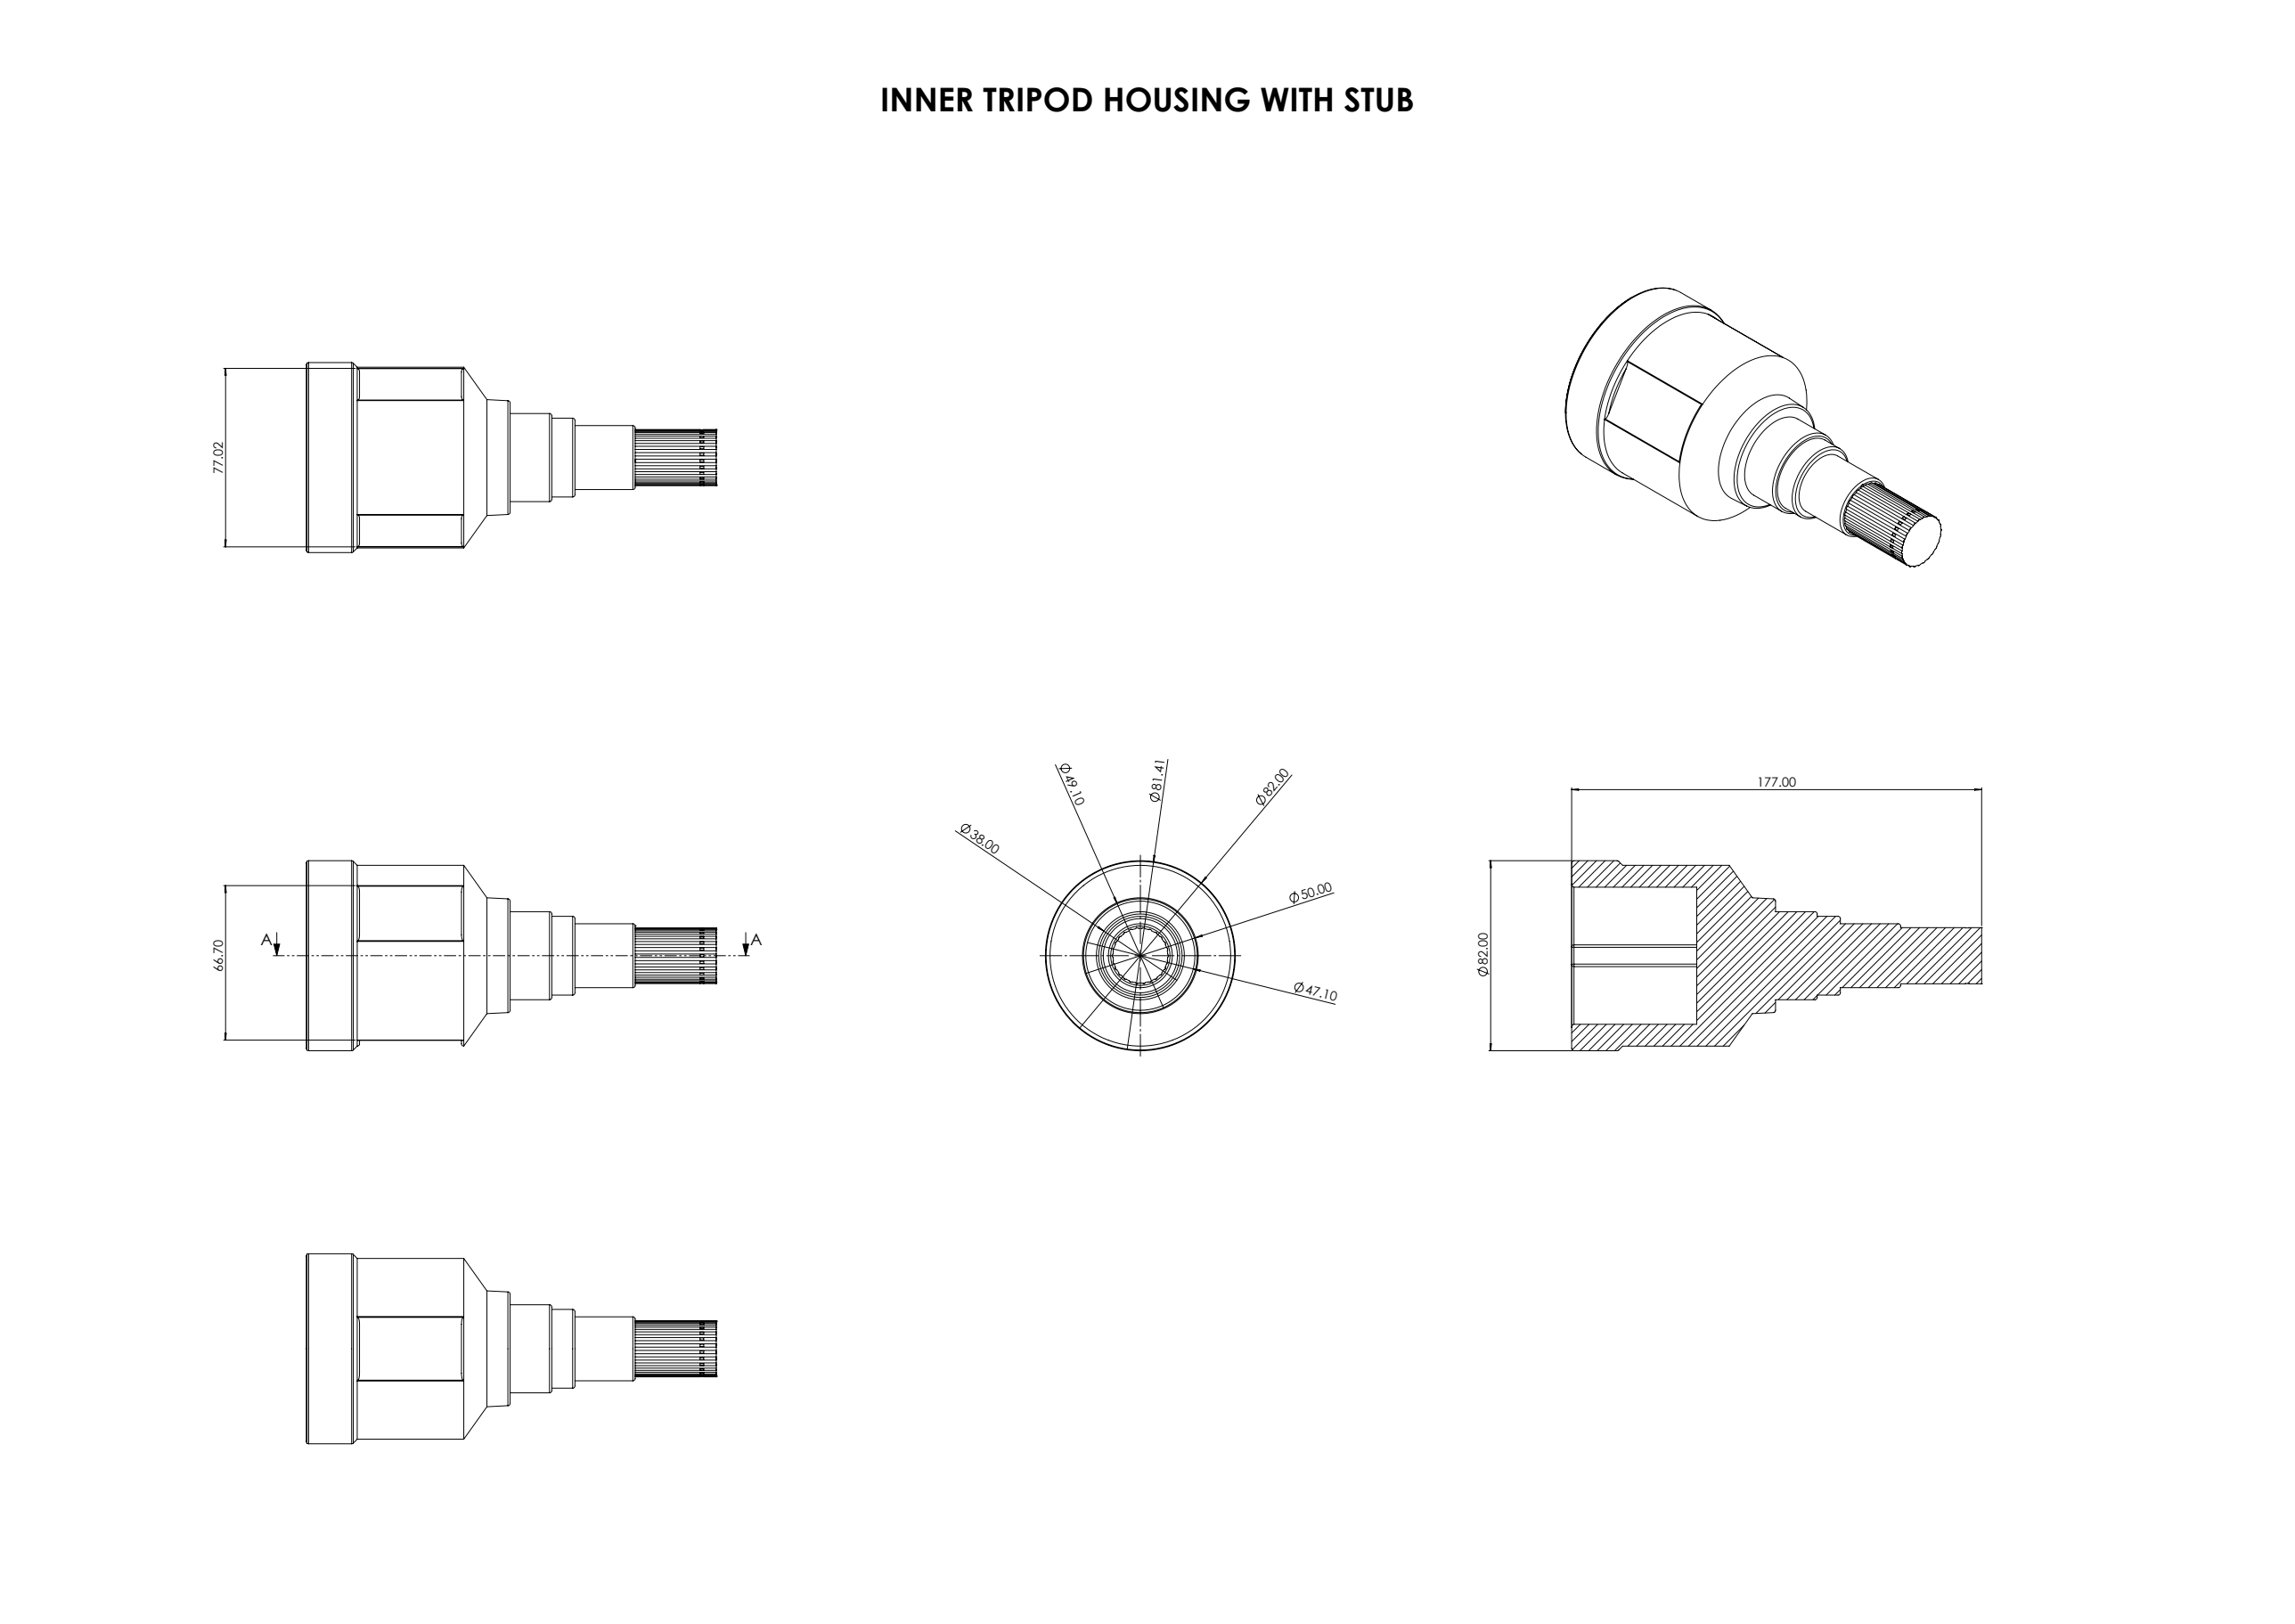
ISO-10303-21;
HEADER;
/* Generated by software containing ST-Developer
 * from STEP Tools, Inc. (www.steptools.com) 
 */

FILE_DESCRIPTION(
/* description */ (''),
/* implementation_level */ '2;1');

FILE_NAME(
/* name */ '13_Inner_Tripod_Housing_with_Stub.step',
/* time_stamp */ '2026-10-11T12:57:03-07:00',
/* author */ (''),
/* organization */ (''),
/* preprocessor_version */ 'ST-DEVELOPER v20.2',
/* originating_system */ 'Autodesk Translation Framework v15.15.0.0',
/* authorisation */ '');

FILE_SCHEMA (('AUTOMOTIVE_DESIGN { 1 0 10303 214 3 1 1 }'));
ENDSEC;

DATA;
#10=MECHANICAL_DESIGN_GEOMETRIC_PRESENTATION_REPRESENTATION('',(#268),#90374);
#234=SHAPE_REPRESENTATION_RELATIONSHIP('SRR','None',#90453,#251);
#251=ADVANCED_BREP_SHAPE_REPRESENTATION('',(#285),#90369);
#268=STYLED_ITEM('',(#90666),#285);
#285=MANIFOLD_SOLID_BREP('Body1',#40357);
#567=SPHERICAL_SURFACE('',#44329,1.);
#568=SPHERICAL_SURFACE('',#44334,1.);
#569=SPHERICAL_SURFACE('',#44356,1.);
#570=SPHERICAL_SURFACE('',#44371,1.);
#571=SPHERICAL_SURFACE('',#44381,1.);
#572=SPHERICAL_SURFACE('',#44386,1.);
#745=CONICAL_SURFACE('',#44294,24.75,0.0499583957219426);
#746=CONICAL_SURFACE('',#44306,40.,0.785398163397441);
#747=CONICAL_SURFACE('',#44318,40.7,0.785398163397426);
#748=CONICAL_SURFACE('',#44512,12.5,0.785398163397459);
#749=CONICAL_SURFACE('',#44524,12.5,0.785398163397459);
#750=CONICAL_SURFACE('',#44534,12.5,0.785398163397459);
#751=CONICAL_SURFACE('',#44544,12.5,0.785398163397459);
#752=CONICAL_SURFACE('',#44554,12.5,0.785398163397459);
#753=CONICAL_SURFACE('',#44564,12.5,0.785398163397459);
#754=CONICAL_SURFACE('',#44574,12.5,0.785398163397459);
#755=CONICAL_SURFACE('',#44584,12.5,0.785398163397459);
#756=CONICAL_SURFACE('',#44594,12.5,0.785398163397459);
#757=CONICAL_SURFACE('',#44604,12.5,0.785398163397459);
#758=CONICAL_SURFACE('',#44614,12.5,0.785398163397459);
#759=CONICAL_SURFACE('',#44624,12.5,0.785398163397459);
#760=CONICAL_SURFACE('',#44634,12.5,0.785398163397459);
#761=CONICAL_SURFACE('',#44644,12.5,0.785398163397459);
#762=CONICAL_SURFACE('',#44654,12.5,0.785398163397459);
#763=CONICAL_SURFACE('',#44664,12.5,0.785398163397459);
#764=CONICAL_SURFACE('',#44674,12.5,0.785398163397459);
#765=CONICAL_SURFACE('',#44684,12.5,0.785398163397459);
#766=CONICAL_SURFACE('',#44694,12.5,0.785398163397459);
#767=CONICAL_SURFACE('',#44704,12.5,0.785398163397459);
#768=CONICAL_SURFACE('',#44714,12.5,0.785398163397459);
#769=CONICAL_SURFACE('',#44724,12.5,0.785398163397459);
#770=CONICAL_SURFACE('',#44734,12.5,0.785398163397459);
#771=CONICAL_SURFACE('',#44744,12.5,0.785398163397459);
#772=CONICAL_SURFACE('',#44750,12.5,0.785398163397459);
#773=CONICAL_SURFACE('',#44773,12.5,0.785398163397459);
#774=CONICAL_SURFACE('',#44807,32.,0.950546840812075);
#991=TOROIDAL_SURFACE('',#44272,16.,1.);
#992=TOROIDAL_SURFACE('',#44281,18.,1.);
#993=TOROIDAL_SURFACE('',#44289,23.548750780275,1.);
#994=TOROIDAL_SURFACE('',#44297,40.,1.);
#995=TOROIDAL_SURFACE('',#44314,40.,1.);
#996=TOROIDAL_SURFACE('',#44324,16.5,1.);
#997=TOROIDAL_SURFACE('',#44339,19.,1.);
#998=TOROIDAL_SURFACE('',#44348,19.,1.);
#999=TOROIDAL_SURFACE('',#44361,16.5,1.);
#1000=TOROIDAL_SURFACE('',#44363,39.9857864376269,1.);
#1001=TOROIDAL_SURFACE('',#44373,16.5,1.);
#1002=TOROIDAL_SURFACE('',#44383,19.,1.);
#1003=TOROIDAL_SURFACE('',#44392,38.,1.);
#1004=TOROIDAL_SURFACE('',#44399,38.,1.);
#1005=TOROIDAL_SURFACE('',#44402,38.,1.);
#1006=TOROIDAL_SURFACE('',#44406,38.,1.);
#1007=TOROIDAL_SURFACE('',#44415,38.,1.);
#1008=TOROIDAL_SURFACE('',#44419,38.,1.);
#1009=TOROIDAL_SURFACE('',#44763,12.8,1.);
#1077=FACE_BOUND('',#6525,.T.);
#1078=FACE_BOUND('',#6529,.T.);
#1079=FACE_BOUND('',#6533,.T.);
#1080=FACE_BOUND('',#6547,.T.);
#1081=FACE_BOUND('',#6588,.T.);
#1082=FACE_BOUND('',#6597,.T.);
#1083=FACE_BOUND('',#6603,.T.);
#1084=FACE_BOUND('',#6609,.T.);
#1085=FACE_BOUND('',#6615,.T.);
#1086=FACE_BOUND('',#6621,.T.);
#1087=FACE_BOUND('',#6627,.T.);
#1088=FACE_BOUND('',#6633,.T.);
#1089=FACE_BOUND('',#6639,.T.);
#1090=FACE_BOUND('',#6645,.T.);
#1091=FACE_BOUND('',#6651,.T.);
#1092=FACE_BOUND('',#6657,.T.);
#1093=FACE_BOUND('',#6663,.T.);
#1094=FACE_BOUND('',#6669,.T.);
#1095=FACE_BOUND('',#6675,.T.);
#1096=FACE_BOUND('',#6681,.T.);
#1097=FACE_BOUND('',#6687,.T.);
#1098=FACE_BOUND('',#6693,.T.);
#1099=FACE_BOUND('',#6699,.T.);
#1100=FACE_BOUND('',#6705,.T.);
#1101=FACE_BOUND('',#6711,.T.);
#1102=FACE_BOUND('',#6717,.T.);
#1103=FACE_BOUND('',#6723,.T.);
#1104=FACE_BOUND('',#6729,.T.);
#1105=FACE_BOUND('',#6735,.T.);
#1106=FACE_BOUND('',#6740,.T.);
#1107=FACE_BOUND('',#6745,.T.);
#1641=PLANE('',#44279);
#1642=PLANE('',#44288);
#1643=PLANE('',#44296);
#1644=PLANE('',#44342);
#1645=PLANE('',#44366);
#1646=PLANE('',#44396);
#1647=PLANE('',#44401);
#1648=PLANE('',#44409);
#1649=PLANE('',#44410);
#1650=PLANE('',#44422);
#1651=PLANE('',#44423);
#1652=PLANE('',#44433);
#1653=PLANE('',#44434);
#1654=PLANE('',#44435);
#1655=PLANE('',#44515);
#1656=PLANE('',#44523);
#1657=PLANE('',#44525);
#1658=PLANE('',#44533);
#1659=PLANE('',#44535);
#1660=PLANE('',#44543);
#1661=PLANE('',#44545);
#1662=PLANE('',#44553);
#1663=PLANE('',#44555);
#1664=PLANE('',#44563);
#1665=PLANE('',#44565);
#1666=PLANE('',#44573);
#1667=PLANE('',#44575);
#1668=PLANE('',#44583);
#1669=PLANE('',#44585);
#1670=PLANE('',#44593);
#1671=PLANE('',#44595);
#1672=PLANE('',#44603);
#1673=PLANE('',#44605);
#1674=PLANE('',#44613);
#1675=PLANE('',#44615);
#1676=PLANE('',#44623);
#1677=PLANE('',#44625);
#1678=PLANE('',#44633);
#1679=PLANE('',#44635);
#1680=PLANE('',#44643);
#1681=PLANE('',#44645);
#1682=PLANE('',#44653);
#1683=PLANE('',#44655);
#1684=PLANE('',#44663);
#1685=PLANE('',#44665);
#1686=PLANE('',#44673);
#1687=PLANE('',#44675);
#1688=PLANE('',#44683);
#1689=PLANE('',#44685);
#1690=PLANE('',#44693);
#1691=PLANE('',#44695);
#1692=PLANE('',#44703);
#1693=PLANE('',#44705);
#1694=PLANE('',#44713);
#1695=PLANE('',#44715);
#1696=PLANE('',#44723);
#1697=PLANE('',#44725);
#1698=PLANE('',#44733);
#1699=PLANE('',#44735);
#1700=PLANE('',#44743);
#1701=PLANE('',#44745);
#1702=PLANE('',#44754);
#1703=PLANE('',#44762);
#1704=PLANE('',#44770);
#1705=PLANE('',#44774);
#1706=PLANE('',#44775);
#1707=PLANE('',#44776);
#1708=PLANE('',#44777);
#1709=PLANE('',#44778);
#1710=PLANE('',#44779);
#1711=PLANE('',#44780);
#1712=PLANE('',#44781);
#1713=PLANE('',#44782);
#1714=PLANE('',#44783);
#1715=PLANE('',#44784);
#1716=PLANE('',#44785);
#1717=PLANE('',#44786);
#1718=PLANE('',#44787);
#1719=PLANE('',#44788);
#1720=PLANE('',#44789);
#1721=PLANE('',#44790);
#1722=PLANE('',#44791);
#1723=PLANE('',#44792);
#1724=PLANE('',#44793);
#1725=PLANE('',#44794);
#1726=PLANE('',#44795);
#1727=PLANE('',#44796);
#1728=PLANE('',#44797);
#1729=PLANE('',#44798);
#1730=PLANE('',#44799);
#1731=PLANE('',#44801);
#1732=PLANE('',#44802);
#1733=PLANE('',#44803);
#1734=PLANE('',#44804);
#1735=PLANE('',#44808);
#4088=FACE_OUTER_BOUND('',#6522,.T.);
#4089=FACE_OUTER_BOUND('',#6523,.T.);
#4090=FACE_OUTER_BOUND('',#6524,.T.);
#4091=FACE_OUTER_BOUND('',#6526,.T.);
#4092=FACE_OUTER_BOUND('',#6527,.T.);
#4093=FACE_OUTER_BOUND('',#6528,.T.);
#4094=FACE_OUTER_BOUND('',#6530,.T.);
#4095=FACE_OUTER_BOUND('',#6531,.T.);
#4096=FACE_OUTER_BOUND('',#6532,.T.);
#4097=FACE_OUTER_BOUND('',#6534,.T.);
#4098=FACE_OUTER_BOUND('',#6535,.T.);
#4099=FACE_OUTER_BOUND('',#6536,.T.);
#4100=FACE_OUTER_BOUND('',#6537,.T.);
#4101=FACE_OUTER_BOUND('',#6538,.T.);
#4102=FACE_OUTER_BOUND('',#6539,.T.);
#4103=FACE_OUTER_BOUND('',#6540,.T.);
#4104=FACE_OUTER_BOUND('',#6541,.T.);
#4105=FACE_OUTER_BOUND('',#6542,.T.);
#4106=FACE_OUTER_BOUND('',#6543,.T.);
#4107=FACE_OUTER_BOUND('',#6544,.T.);
#4108=FACE_OUTER_BOUND('',#6545,.T.);
#4109=FACE_OUTER_BOUND('',#6546,.T.);
#4110=FACE_OUTER_BOUND('',#6548,.T.);
#4111=FACE_OUTER_BOUND('',#6549,.T.);
#4112=FACE_OUTER_BOUND('',#6550,.T.);
#4113=FACE_OUTER_BOUND('',#6551,.T.);
#4114=FACE_OUTER_BOUND('',#6552,.T.);
#4115=FACE_OUTER_BOUND('',#6553,.T.);
#4116=FACE_OUTER_BOUND('',#6554,.T.);
#4117=FACE_OUTER_BOUND('',#6555,.T.);
#4118=FACE_OUTER_BOUND('',#6556,.T.);
#4119=FACE_OUTER_BOUND('',#6557,.T.);
#4120=FACE_OUTER_BOUND('',#6558,.T.);
#4121=FACE_OUTER_BOUND('',#6559,.T.);
#4122=FACE_OUTER_BOUND('',#6560,.T.);
#4123=FACE_OUTER_BOUND('',#6561,.T.);
#4124=FACE_OUTER_BOUND('',#6562,.T.);
#4125=FACE_OUTER_BOUND('',#6563,.T.);
#4126=FACE_OUTER_BOUND('',#6564,.T.);
#4127=FACE_OUTER_BOUND('',#6565,.T.);
#4128=FACE_OUTER_BOUND('',#6566,.T.);
#4129=FACE_OUTER_BOUND('',#6567,.T.);
#4130=FACE_OUTER_BOUND('',#6568,.T.);
#4131=FACE_OUTER_BOUND('',#6569,.T.);
#4132=FACE_OUTER_BOUND('',#6570,.T.);
#4133=FACE_OUTER_BOUND('',#6571,.T.);
#4134=FACE_OUTER_BOUND('',#6572,.T.);
#4135=FACE_OUTER_BOUND('',#6573,.T.);
#4136=FACE_OUTER_BOUND('',#6574,.T.);
#4137=FACE_OUTER_BOUND('',#6575,.T.);
#4138=FACE_OUTER_BOUND('',#6576,.T.);
#4139=FACE_OUTER_BOUND('',#6577,.T.);
#4140=FACE_OUTER_BOUND('',#6578,.T.);
#4141=FACE_OUTER_BOUND('',#6579,.T.);
#4142=FACE_OUTER_BOUND('',#6580,.T.);
#4143=FACE_OUTER_BOUND('',#6581,.T.);
#4144=FACE_OUTER_BOUND('',#6582,.T.);
#4145=FACE_OUTER_BOUND('',#6583,.T.);
#4146=FACE_OUTER_BOUND('',#6584,.T.);
#4147=FACE_OUTER_BOUND('',#6585,.T.);
#4148=FACE_OUTER_BOUND('',#6586,.T.);
#4149=FACE_OUTER_BOUND('',#6587,.T.);
#4150=FACE_OUTER_BOUND('',#6589,.T.);
#4151=FACE_OUTER_BOUND('',#6590,.T.);
#4152=FACE_OUTER_BOUND('',#6591,.T.);
#4153=FACE_OUTER_BOUND('',#6592,.T.);
#4154=FACE_OUTER_BOUND('',#6593,.T.);
#4155=FACE_OUTER_BOUND('',#6594,.T.);
#4156=FACE_OUTER_BOUND('',#6595,.T.);
#4157=FACE_OUTER_BOUND('',#6596,.T.);
#4158=FACE_OUTER_BOUND('',#6598,.T.);
#4159=FACE_OUTER_BOUND('',#6599,.T.);
#4160=FACE_OUTER_BOUND('',#6600,.T.);
#4161=FACE_OUTER_BOUND('',#6601,.T.);
#4162=FACE_OUTER_BOUND('',#6602,.T.);
#4163=FACE_OUTER_BOUND('',#6604,.T.);
#4164=FACE_OUTER_BOUND('',#6605,.T.);
#4165=FACE_OUTER_BOUND('',#6606,.T.);
#4166=FACE_OUTER_BOUND('',#6607,.T.);
#4167=FACE_OUTER_BOUND('',#6608,.T.);
#4168=FACE_OUTER_BOUND('',#6610,.T.);
#4169=FACE_OUTER_BOUND('',#6611,.T.);
#4170=FACE_OUTER_BOUND('',#6612,.T.);
#4171=FACE_OUTER_BOUND('',#6613,.T.);
#4172=FACE_OUTER_BOUND('',#6614,.T.);
#4173=FACE_OUTER_BOUND('',#6616,.T.);
#4174=FACE_OUTER_BOUND('',#6617,.T.);
#4175=FACE_OUTER_BOUND('',#6618,.T.);
#4176=FACE_OUTER_BOUND('',#6619,.T.);
#4177=FACE_OUTER_BOUND('',#6620,.T.);
#4178=FACE_OUTER_BOUND('',#6622,.T.);
#4179=FACE_OUTER_BOUND('',#6623,.T.);
#4180=FACE_OUTER_BOUND('',#6624,.T.);
#4181=FACE_OUTER_BOUND('',#6625,.T.);
#4182=FACE_OUTER_BOUND('',#6626,.T.);
#4183=FACE_OUTER_BOUND('',#6628,.T.);
#4184=FACE_OUTER_BOUND('',#6629,.T.);
#4185=FACE_OUTER_BOUND('',#6630,.T.);
#4186=FACE_OUTER_BOUND('',#6631,.T.);
#4187=FACE_OUTER_BOUND('',#6632,.T.);
#4188=FACE_OUTER_BOUND('',#6634,.T.);
#4189=FACE_OUTER_BOUND('',#6635,.T.);
#4190=FACE_OUTER_BOUND('',#6636,.T.);
#4191=FACE_OUTER_BOUND('',#6637,.T.);
#4192=FACE_OUTER_BOUND('',#6638,.T.);
#4193=FACE_OUTER_BOUND('',#6640,.T.);
#4194=FACE_OUTER_BOUND('',#6641,.T.);
#4195=FACE_OUTER_BOUND('',#6642,.T.);
#4196=FACE_OUTER_BOUND('',#6643,.T.);
#4197=FACE_OUTER_BOUND('',#6644,.T.);
#4198=FACE_OUTER_BOUND('',#6646,.T.);
#4199=FACE_OUTER_BOUND('',#6647,.T.);
#4200=FACE_OUTER_BOUND('',#6648,.T.);
#4201=FACE_OUTER_BOUND('',#6649,.T.);
#4202=FACE_OUTER_BOUND('',#6650,.T.);
#4203=FACE_OUTER_BOUND('',#6652,.T.);
#4204=FACE_OUTER_BOUND('',#6653,.T.);
#4205=FACE_OUTER_BOUND('',#6654,.T.);
#4206=FACE_OUTER_BOUND('',#6655,.T.);
#4207=FACE_OUTER_BOUND('',#6656,.T.);
#4208=FACE_OUTER_BOUND('',#6658,.T.);
#4209=FACE_OUTER_BOUND('',#6659,.T.);
#4210=FACE_OUTER_BOUND('',#6660,.T.);
#4211=FACE_OUTER_BOUND('',#6661,.T.);
#4212=FACE_OUTER_BOUND('',#6662,.T.);
#4213=FACE_OUTER_BOUND('',#6664,.T.);
#4214=FACE_OUTER_BOUND('',#6665,.T.);
#4215=FACE_OUTER_BOUND('',#6666,.T.);
#4216=FACE_OUTER_BOUND('',#6667,.T.);
#4217=FACE_OUTER_BOUND('',#6668,.T.);
#4218=FACE_OUTER_BOUND('',#6670,.T.);
#4219=FACE_OUTER_BOUND('',#6671,.T.);
#4220=FACE_OUTER_BOUND('',#6672,.T.);
#4221=FACE_OUTER_BOUND('',#6673,.T.);
#4222=FACE_OUTER_BOUND('',#6674,.T.);
#4223=FACE_OUTER_BOUND('',#6676,.T.);
#4224=FACE_OUTER_BOUND('',#6677,.T.);
#4225=FACE_OUTER_BOUND('',#6678,.T.);
#4226=FACE_OUTER_BOUND('',#6679,.T.);
#4227=FACE_OUTER_BOUND('',#6680,.T.);
#4228=FACE_OUTER_BOUND('',#6682,.T.);
#4229=FACE_OUTER_BOUND('',#6683,.T.);
#4230=FACE_OUTER_BOUND('',#6684,.T.);
#4231=FACE_OUTER_BOUND('',#6685,.T.);
#4232=FACE_OUTER_BOUND('',#6686,.T.);
#4233=FACE_OUTER_BOUND('',#6688,.T.);
#4234=FACE_OUTER_BOUND('',#6689,.T.);
#4235=FACE_OUTER_BOUND('',#6690,.T.);
#4236=FACE_OUTER_BOUND('',#6691,.T.);
#4237=FACE_OUTER_BOUND('',#6692,.T.);
#4238=FACE_OUTER_BOUND('',#6694,.T.);
#4239=FACE_OUTER_BOUND('',#6695,.T.);
#4240=FACE_OUTER_BOUND('',#6696,.T.);
#4241=FACE_OUTER_BOUND('',#6697,.T.);
#4242=FACE_OUTER_BOUND('',#6698,.T.);
#4243=FACE_OUTER_BOUND('',#6700,.T.);
#4244=FACE_OUTER_BOUND('',#6701,.T.);
#4245=FACE_OUTER_BOUND('',#6702,.T.);
#4246=FACE_OUTER_BOUND('',#6703,.T.);
#4247=FACE_OUTER_BOUND('',#6704,.T.);
#4248=FACE_OUTER_BOUND('',#6706,.T.);
#4249=FACE_OUTER_BOUND('',#6707,.T.);
#4250=FACE_OUTER_BOUND('',#6708,.T.);
#4251=FACE_OUTER_BOUND('',#6709,.T.);
#4252=FACE_OUTER_BOUND('',#6710,.T.);
#4253=FACE_OUTER_BOUND('',#6712,.T.);
#4254=FACE_OUTER_BOUND('',#6713,.T.);
#4255=FACE_OUTER_BOUND('',#6714,.T.);
#4256=FACE_OUTER_BOUND('',#6715,.T.);
#4257=FACE_OUTER_BOUND('',#6716,.T.);
#4258=FACE_OUTER_BOUND('',#6718,.T.);
#4259=FACE_OUTER_BOUND('',#6719,.T.);
#4260=FACE_OUTER_BOUND('',#6720,.T.);
#4261=FACE_OUTER_BOUND('',#6721,.T.);
#4262=FACE_OUTER_BOUND('',#6722,.T.);
#4263=FACE_OUTER_BOUND('',#6724,.T.);
#4264=FACE_OUTER_BOUND('',#6725,.T.);
#4265=FACE_OUTER_BOUND('',#6726,.T.);
#4266=FACE_OUTER_BOUND('',#6727,.T.);
#4267=FACE_OUTER_BOUND('',#6728,.T.);
#4268=FACE_OUTER_BOUND('',#6730,.T.);
#4269=FACE_OUTER_BOUND('',#6731,.T.);
#4270=FACE_OUTER_BOUND('',#6732,.T.);
#4271=FACE_OUTER_BOUND('',#6733,.T.);
#4272=FACE_OUTER_BOUND('',#6734,.T.);
#4273=FACE_OUTER_BOUND('',#6736,.T.);
#4274=FACE_OUTER_BOUND('',#6737,.T.);
#4275=FACE_OUTER_BOUND('',#6738,.T.);
#4276=FACE_OUTER_BOUND('',#6739,.T.);
#4277=FACE_OUTER_BOUND('',#6741,.T.);
#4278=FACE_OUTER_BOUND('',#6742,.T.);
#4279=FACE_OUTER_BOUND('',#6743,.T.);
#4280=FACE_OUTER_BOUND('',#6744,.T.);
#4281=FACE_OUTER_BOUND('',#6746,.T.);
#4282=FACE_OUTER_BOUND('',#6747,.T.);
#4283=FACE_OUTER_BOUND('',#6748,.T.);
#4284=FACE_OUTER_BOUND('',#6749,.T.);
#4285=FACE_OUTER_BOUND('',#6750,.T.);
#4286=FACE_OUTER_BOUND('',#6751,.T.);
#4287=FACE_OUTER_BOUND('',#6752,.T.);
#4288=FACE_OUTER_BOUND('',#6753,.T.);
#4289=FACE_OUTER_BOUND('',#6754,.T.);
#4290=FACE_OUTER_BOUND('',#6755,.T.);
#4291=FACE_OUTER_BOUND('',#6756,.T.);
#4292=FACE_OUTER_BOUND('',#6757,.T.);
#4293=FACE_OUTER_BOUND('',#6758,.T.);
#4294=FACE_OUTER_BOUND('',#6759,.T.);
#4295=FACE_OUTER_BOUND('',#6760,.T.);
#4296=FACE_OUTER_BOUND('',#6761,.T.);
#4297=FACE_OUTER_BOUND('',#6762,.T.);
#4298=FACE_OUTER_BOUND('',#6763,.T.);
#4299=FACE_OUTER_BOUND('',#6764,.T.);
#4300=FACE_OUTER_BOUND('',#6765,.T.);
#4301=FACE_OUTER_BOUND('',#6766,.T.);
#4302=FACE_OUTER_BOUND('',#6767,.T.);
#4303=FACE_OUTER_BOUND('',#6768,.T.);
#4304=FACE_OUTER_BOUND('',#6769,.T.);
#4305=FACE_OUTER_BOUND('',#6770,.T.);
#4306=FACE_OUTER_BOUND('',#6771,.T.);
#4307=FACE_OUTER_BOUND('',#6772,.T.);
#4308=FACE_OUTER_BOUND('',#6773,.T.);
#4309=FACE_OUTER_BOUND('',#6774,.T.);
#4310=FACE_OUTER_BOUND('',#6775,.T.);
#4311=FACE_OUTER_BOUND('',#6776,.T.);
#4312=FACE_OUTER_BOUND('',#6777,.T.);
#4313=FACE_OUTER_BOUND('',#6778,.T.);
#4314=FACE_OUTER_BOUND('',#6779,.T.);
#4315=FACE_OUTER_BOUND('',#6780,.T.);
#4316=FACE_OUTER_BOUND('',#6781,.T.);
#6522=EDGE_LOOP('',(#34861,#34862,#34863,#34864,#34865));
#6523=EDGE_LOOP('',(#34866,#34867,#34868,#34869,#34870));
#6524=EDGE_LOOP('',(#34871));
#6525=EDGE_LOOP('',(#34872));
#6526=EDGE_LOOP('',(#34873,#34874,#34875,#34876,#34877));
#6527=EDGE_LOOP('',(#34878,#34879,#34880,#34881,#34882));
#6528=EDGE_LOOP('',(#34883));
#6529=EDGE_LOOP('',(#34884));
#6530=EDGE_LOOP('',(#34885,#34886,#34887,#34888,#34889));
#6531=EDGE_LOOP('',(#34890,#34891,#34892,#34893,#34894));
#6532=EDGE_LOOP('',(#34895));
#6533=EDGE_LOOP('',(#34896));
#6534=EDGE_LOOP('',(#34897,#34898,#34899,#34900,#34901,#34902));
#6535=EDGE_LOOP('',(#34903,#34904,#34905,#34906,#34907,#34908));
#6536=EDGE_LOOP('',(#34909,#34910,#34911,#34912,#34913,#34914,#34915,#34916,
#34917,#34918,#34919));
#6537=EDGE_LOOP('',(#34920,#34921,#34922,#34923,#34924,#34925));
#6538=EDGE_LOOP('',(#34926,#34927,#34928,#34929,#34930,#34931));
#6539=EDGE_LOOP('',(#34932,#34933,#34934,#34935));
#6540=EDGE_LOOP('',(#34936,#34937,#34938,#34939));
#6541=EDGE_LOOP('',(#34940,#34941,#34942));
#6542=EDGE_LOOP('',(#34943,#34944,#34945,#34946));
#6543=EDGE_LOOP('',(#34947,#34948,#34949));
#6544=EDGE_LOOP('',(#34950,#34951,#34952,#34953));
#6545=EDGE_LOOP('',(#34954,#34955,#34956,#34957));
#6546=EDGE_LOOP('',(#34958));
#6547=EDGE_LOOP('',(#34959,#34960,#34961,#34962,#34963,#34964));
#6548=EDGE_LOOP('',(#34965,#34966,#34967,#34968));
#6549=EDGE_LOOP('',(#34969,#34970,#34971,#34972));
#6550=EDGE_LOOP('',(#34973,#34974,#34975,#34976));
#6551=EDGE_LOOP('',(#34977,#34978,#34979));
#6552=EDGE_LOOP('',(#34980,#34981,#34982,#34983));
#6553=EDGE_LOOP('',(#34984,#34985,#34986,#34987));
#6554=EDGE_LOOP('',(#34988,#34989,#34990,#34991,#34992));
#6555=EDGE_LOOP('',(#34993,#34994,#34995,#34996));
#6556=EDGE_LOOP('',(#34997,#34998,#34999,#35000,#35001,#35002,#35003,#35004));
#6557=EDGE_LOOP('',(#35005,#35006,#35007,#35008));
#6558=EDGE_LOOP('',(#35009,#35010,#35011,#35012));
#6559=EDGE_LOOP('',(#35013,#35014,#35015));
#6560=EDGE_LOOP('',(#35016,#35017,#35018,#35019));
#6561=EDGE_LOOP('',(#35020,#35021,#35022,#35023));
#6562=EDGE_LOOP('',(#35024,#35025,#35026,#35027));
#6563=EDGE_LOOP('',(#35028,#35029,#35030));
#6564=EDGE_LOOP('',(#35031,#35032,#35033,#35034));
#6565=EDGE_LOOP('',(#35035,#35036,#35037));
#6566=EDGE_LOOP('',(#35038,#35039,#35040,#35041));
#6567=EDGE_LOOP('',(#35042,#35043,#35044,#35045));
#6568=EDGE_LOOP('',(#35046,#35047,#35048,#35049,#35050,#35051,#35052));
#6569=EDGE_LOOP('',(#35053,#35054));
#6570=EDGE_LOOP('',(#35055,#35056,#35057,#35058));
#6571=EDGE_LOOP('',(#35059,#35060,#35061,#35062,#35063,#35064,#35065));
#6572=EDGE_LOOP('',(#35066,#35067));
#6573=EDGE_LOOP('',(#35068,#35069,#35070,#35071,#35072,#35073));
#6574=EDGE_LOOP('',(#35074,#35075,#35076,#35077));
#6575=EDGE_LOOP('',(#35078,#35079,#35080,#35081));
#6576=EDGE_LOOP('',(#35082,#35083,#35084,#35085,#35086,#35087));
#6577=EDGE_LOOP('',(#35088,#35089,#35090,#35091,#35092,#35093,#35094,#35095));
#6578=EDGE_LOOP('',(#35096,#35097));
#6579=EDGE_LOOP('',(#35098,#35099,#35100,#35101));
#6580=EDGE_LOOP('',(#35102,#35103,#35104,#35105));
#6581=EDGE_LOOP('',(#35106,#35107,#35108,#35109,#35110,#35111));
#6582=EDGE_LOOP('',(#35112,#35113,#35114,#35115));
#6583=EDGE_LOOP('',(#35116,#35117,#35118,#35119));
#6584=EDGE_LOOP('',(#35120,#35121,#35122,#35123,#35124,#35125));
#6585=EDGE_LOOP('',(#35126,#35127,#35128,#35129,#35130,#35131,#35132,#35133));
#6586=EDGE_LOOP('',(#35134,#35135));
#6587=EDGE_LOOP('',(#35136,#35137,#35138,#35139,#35140,#35141));
#6588=EDGE_LOOP('',(#35142,#35143,#35144,#35145));
#6589=EDGE_LOOP('',(#35146,#35147,#35148,#35149));
#6590=EDGE_LOOP('',(#35150,#35151));
#6591=EDGE_LOOP('',(#35152,#35153,#35154));
#6592=EDGE_LOOP('',(#35155,#35156,#35157,#35158,#35159,#35160,#35161,#35162,
#35163,#35164,#35165,#35166,#35167,#35168,#35169,#35170,#35171,#35172,#35173,
#35174,#35175,#35176,#35177,#35178,#35179,#35180,#35181,#35182,#35183,#35184,
#35185,#35186,#35187,#35188,#35189,#35190,#35191,#35192,#35193,#35194,#35195,
#35196,#35197,#35198,#35199,#35200,#35201,#35202,#35203,#35204,#35205,#35206,
#35207,#35208,#35209,#35210,#35211,#35212,#35213,#35214,#35215,#35216,#35217,
#35218,#35219,#35220,#35221,#35222,#35223,#35224,#35225,#35226,#35227,#35228,
#35229,#35230,#35231,#35232,#35233,#35234,#35235,#35236,#35237,#35238,#35239,
#35240,#35241,#35242,#35243,#35244,#35245,#35246,#35247,#35248,#35249,#35250,
#35251,#35252,#35253,#35254,#35255,#35256,#35257,#35258));
#6593=EDGE_LOOP('',(#35259,#35260));
#6594=EDGE_LOOP('',(#35261,#35262,#35263));
#6595=EDGE_LOOP('',(#35264,#35265));
#6596=EDGE_LOOP('',(#35266,#35267,#35268,#35269,#35270,#35271));
#6597=EDGE_LOOP('',(#35272,#35273,#35274,#35275));
#6598=EDGE_LOOP('',(#35276,#35277,#35278,#35279));
#6599=EDGE_LOOP('',(#35280,#35281));
#6600=EDGE_LOOP('',(#35282,#35283));
#6601=EDGE_LOOP('',(#35284,#35285));
#6602=EDGE_LOOP('',(#35286,#35287,#35288,#35289,#35290,#35291));
#6603=EDGE_LOOP('',(#35292,#35293,#35294,#35295));
#6604=EDGE_LOOP('',(#35296,#35297,#35298,#35299));
#6605=EDGE_LOOP('',(#35300,#35301));
#6606=EDGE_LOOP('',(#35302,#35303));
#6607=EDGE_LOOP('',(#35304,#35305));
#6608=EDGE_LOOP('',(#35306,#35307,#35308,#35309,#35310,#35311));
#6609=EDGE_LOOP('',(#35312,#35313,#35314,#35315));
#6610=EDGE_LOOP('',(#35316,#35317,#35318,#35319));
#6611=EDGE_LOOP('',(#35320,#35321));
#6612=EDGE_LOOP('',(#35322,#35323));
#6613=EDGE_LOOP('',(#35324,#35325));
#6614=EDGE_LOOP('',(#35326,#35327,#35328,#35329,#35330,#35331));
#6615=EDGE_LOOP('',(#35332,#35333,#35334,#35335));
#6616=EDGE_LOOP('',(#35336,#35337,#35338,#35339));
#6617=EDGE_LOOP('',(#35340,#35341));
#6618=EDGE_LOOP('',(#35342,#35343));
#6619=EDGE_LOOP('',(#35344,#35345));
#6620=EDGE_LOOP('',(#35346,#35347,#35348,#35349,#35350,#35351));
#6621=EDGE_LOOP('',(#35352,#35353,#35354,#35355));
#6622=EDGE_LOOP('',(#35356,#35357,#35358,#35359));
#6623=EDGE_LOOP('',(#35360,#35361));
#6624=EDGE_LOOP('',(#35362,#35363));
#6625=EDGE_LOOP('',(#35364,#35365));
#6626=EDGE_LOOP('',(#35366,#35367,#35368,#35369,#35370,#35371));
#6627=EDGE_LOOP('',(#35372,#35373,#35374,#35375));
#6628=EDGE_LOOP('',(#35376,#35377,#35378,#35379));
#6629=EDGE_LOOP('',(#35380,#35381));
#6630=EDGE_LOOP('',(#35382,#35383));
#6631=EDGE_LOOP('',(#35384,#35385));
#6632=EDGE_LOOP('',(#35386,#35387,#35388,#35389,#35390,#35391));
#6633=EDGE_LOOP('',(#35392,#35393,#35394,#35395));
#6634=EDGE_LOOP('',(#35396,#35397,#35398,#35399));
#6635=EDGE_LOOP('',(#35400,#35401));
#6636=EDGE_LOOP('',(#35402,#35403));
#6637=EDGE_LOOP('',(#35404,#35405));
#6638=EDGE_LOOP('',(#35406,#35407,#35408,#35409,#35410,#35411));
#6639=EDGE_LOOP('',(#35412,#35413,#35414,#35415));
#6640=EDGE_LOOP('',(#35416,#35417,#35418,#35419));
#6641=EDGE_LOOP('',(#35420,#35421));
#6642=EDGE_LOOP('',(#35422,#35423));
#6643=EDGE_LOOP('',(#35424,#35425));
#6644=EDGE_LOOP('',(#35426,#35427,#35428,#35429,#35430,#35431));
#6645=EDGE_LOOP('',(#35432,#35433,#35434,#35435));
#6646=EDGE_LOOP('',(#35436,#35437,#35438,#35439));
#6647=EDGE_LOOP('',(#35440,#35441));
#6648=EDGE_LOOP('',(#35442,#35443));
#6649=EDGE_LOOP('',(#35444,#35445));
#6650=EDGE_LOOP('',(#35446,#35447,#35448,#35449,#35450,#35451));
#6651=EDGE_LOOP('',(#35452,#35453,#35454,#35455));
#6652=EDGE_LOOP('',(#35456,#35457,#35458,#35459));
#6653=EDGE_LOOP('',(#35460,#35461));
#6654=EDGE_LOOP('',(#35462,#35463));
#6655=EDGE_LOOP('',(#35464,#35465));
#6656=EDGE_LOOP('',(#35466,#35467,#35468,#35469,#35470,#35471));
#6657=EDGE_LOOP('',(#35472,#35473,#35474,#35475));
#6658=EDGE_LOOP('',(#35476,#35477,#35478,#35479));
#6659=EDGE_LOOP('',(#35480,#35481));
#6660=EDGE_LOOP('',(#35482,#35483));
#6661=EDGE_LOOP('',(#35484,#35485));
#6662=EDGE_LOOP('',(#35486,#35487,#35488,#35489,#35490,#35491));
#6663=EDGE_LOOP('',(#35492,#35493,#35494,#35495));
#6664=EDGE_LOOP('',(#35496,#35497,#35498,#35499));
#6665=EDGE_LOOP('',(#35500,#35501));
#6666=EDGE_LOOP('',(#35502,#35503));
#6667=EDGE_LOOP('',(#35504,#35505));
#6668=EDGE_LOOP('',(#35506,#35507,#35508,#35509,#35510,#35511));
#6669=EDGE_LOOP('',(#35512,#35513,#35514,#35515));
#6670=EDGE_LOOP('',(#35516,#35517,#35518,#35519));
#6671=EDGE_LOOP('',(#35520,#35521));
#6672=EDGE_LOOP('',(#35522,#35523));
#6673=EDGE_LOOP('',(#35524,#35525));
#6674=EDGE_LOOP('',(#35526,#35527,#35528,#35529,#35530,#35531));
#6675=EDGE_LOOP('',(#35532,#35533,#35534,#35535));
#6676=EDGE_LOOP('',(#35536,#35537,#35538,#35539));
#6677=EDGE_LOOP('',(#35540,#35541));
#6678=EDGE_LOOP('',(#35542,#35543));
#6679=EDGE_LOOP('',(#35544,#35545));
#6680=EDGE_LOOP('',(#35546,#35547,#35548,#35549,#35550,#35551));
#6681=EDGE_LOOP('',(#35552,#35553,#35554,#35555));
#6682=EDGE_LOOP('',(#35556,#35557,#35558,#35559));
#6683=EDGE_LOOP('',(#35560,#35561));
#6684=EDGE_LOOP('',(#35562,#35563));
#6685=EDGE_LOOP('',(#35564,#35565));
#6686=EDGE_LOOP('',(#35566,#35567,#35568,#35569,#35570,#35571));
#6687=EDGE_LOOP('',(#35572,#35573,#35574,#35575));
#6688=EDGE_LOOP('',(#35576,#35577,#35578,#35579));
#6689=EDGE_LOOP('',(#35580,#35581));
#6690=EDGE_LOOP('',(#35582,#35583));
#6691=EDGE_LOOP('',(#35584,#35585));
#6692=EDGE_LOOP('',(#35586,#35587,#35588,#35589,#35590,#35591));
#6693=EDGE_LOOP('',(#35592,#35593,#35594,#35595));
#6694=EDGE_LOOP('',(#35596,#35597,#35598,#35599));
#6695=EDGE_LOOP('',(#35600,#35601));
#6696=EDGE_LOOP('',(#35602,#35603));
#6697=EDGE_LOOP('',(#35604,#35605));
#6698=EDGE_LOOP('',(#35606,#35607,#35608,#35609,#35610,#35611));
#6699=EDGE_LOOP('',(#35612,#35613,#35614,#35615));
#6700=EDGE_LOOP('',(#35616,#35617,#35618,#35619));
#6701=EDGE_LOOP('',(#35620,#35621));
#6702=EDGE_LOOP('',(#35622,#35623));
#6703=EDGE_LOOP('',(#35624,#35625));
#6704=EDGE_LOOP('',(#35626,#35627,#35628,#35629,#35630,#35631));
#6705=EDGE_LOOP('',(#35632,#35633,#35634,#35635));
#6706=EDGE_LOOP('',(#35636,#35637,#35638,#35639));
#6707=EDGE_LOOP('',(#35640,#35641));
#6708=EDGE_LOOP('',(#35642,#35643));
#6709=EDGE_LOOP('',(#35644,#35645));
#6710=EDGE_LOOP('',(#35646,#35647,#35648,#35649,#35650,#35651));
#6711=EDGE_LOOP('',(#35652,#35653,#35654,#35655));
#6712=EDGE_LOOP('',(#35656,#35657,#35658,#35659));
#6713=EDGE_LOOP('',(#35660,#35661));
#6714=EDGE_LOOP('',(#35662,#35663));
#6715=EDGE_LOOP('',(#35664,#35665));
#6716=EDGE_LOOP('',(#35666,#35667,#35668,#35669,#35670,#35671));
#6717=EDGE_LOOP('',(#35672,#35673,#35674,#35675));
#6718=EDGE_LOOP('',(#35676,#35677,#35678,#35679));
#6719=EDGE_LOOP('',(#35680,#35681));
#6720=EDGE_LOOP('',(#35682,#35683));
#6721=EDGE_LOOP('',(#35684,#35685));
#6722=EDGE_LOOP('',(#35686,#35687,#35688,#35689,#35690,#35691));
#6723=EDGE_LOOP('',(#35692,#35693,#35694,#35695));
#6724=EDGE_LOOP('',(#35696,#35697,#35698,#35699));
#6725=EDGE_LOOP('',(#35700,#35701));
#6726=EDGE_LOOP('',(#35702,#35703));
#6727=EDGE_LOOP('',(#35704,#35705));
#6728=EDGE_LOOP('',(#35706,#35707,#35708,#35709,#35710,#35711));
#6729=EDGE_LOOP('',(#35712,#35713,#35714,#35715));
#6730=EDGE_LOOP('',(#35716,#35717,#35718,#35719));
#6731=EDGE_LOOP('',(#35720,#35721));
#6732=EDGE_LOOP('',(#35722,#35723));
#6733=EDGE_LOOP('',(#35724,#35725));
#6734=EDGE_LOOP('',(#35726,#35727,#35728,#35729,#35730,#35731));
#6735=EDGE_LOOP('',(#35732,#35733,#35734,#35735));
#6736=EDGE_LOOP('',(#35736,#35737));
#6737=EDGE_LOOP('',(#35738,#35739,#35740,#35741));
#6738=EDGE_LOOP('',(#35742,#35743));
#6739=EDGE_LOOP('',(#35744,#35745,#35746,#35747,#35748,#35749));
#6740=EDGE_LOOP('',(#35750,#35751,#35752,#35753));
#6741=EDGE_LOOP('',(#35754,#35755,#35756,#35757));
#6742=EDGE_LOOP('',(#35758,#35759));
#6743=EDGE_LOOP('',(#35760,#35761,#35762,#35763,#35764,#35765,#35766,#35767,
#35768));
#6744=EDGE_LOOP('',(#35769,#35770,#35771,#35772,#35773));
#6745=EDGE_LOOP('',(#35774,#35775,#35776,#35777,#35778,#35779,#35780,#35781,
#35782,#35783,#35784,#35785,#35786,#35787,#35788,#35789,#35790,#35791,#35792,
#35793,#35794,#35795,#35796,#35797,#35798,#35799,#35800,#35801,#35802,#35803,
#35804,#35805,#35806,#35807,#35808,#35809,#35810,#35811,#35812,#35813,#35814,
#35815,#35816,#35817,#35818,#35819,#35820,#35821,#35822,#35823,#35824,#35825));
#6746=EDGE_LOOP('',(#35826,#35827,#35828,#35829,#35830));
#6747=EDGE_LOOP('',(#35831,#35832));
#6748=EDGE_LOOP('',(#35833,#35834,#35835,#35836));
#6749=EDGE_LOOP('',(#35837,#35838));
#6750=EDGE_LOOP('',(#35839,#35840,#35841,#35842));
#6751=EDGE_LOOP('',(#35843,#35844,#35845,#35846));
#6752=EDGE_LOOP('',(#35847,#35848,#35849,#35850));
#6753=EDGE_LOOP('',(#35851,#35852,#35853,#35854));
#6754=EDGE_LOOP('',(#35855,#35856,#35857,#35858));
#6755=EDGE_LOOP('',(#35859,#35860,#35861,#35862));
#6756=EDGE_LOOP('',(#35863,#35864,#35865,#35866));
#6757=EDGE_LOOP('',(#35867,#35868,#35869,#35870));
#6758=EDGE_LOOP('',(#35871,#35872,#35873,#35874));
#6759=EDGE_LOOP('',(#35875,#35876,#35877,#35878));
#6760=EDGE_LOOP('',(#35879,#35880,#35881,#35882));
#6761=EDGE_LOOP('',(#35883,#35884,#35885,#35886));
#6762=EDGE_LOOP('',(#35887,#35888,#35889,#35890));
#6763=EDGE_LOOP('',(#35891,#35892,#35893,#35894));
#6764=EDGE_LOOP('',(#35895,#35896,#35897,#35898));
#6765=EDGE_LOOP('',(#35899,#35900,#35901,#35902));
#6766=EDGE_LOOP('',(#35903,#35904,#35905,#35906));
#6767=EDGE_LOOP('',(#35907,#35908,#35909,#35910));
#6768=EDGE_LOOP('',(#35911,#35912,#35913,#35914));
#6769=EDGE_LOOP('',(#35915,#35916,#35917,#35918));
#6770=EDGE_LOOP('',(#35919,#35920,#35921,#35922));
#6771=EDGE_LOOP('',(#35923,#35924,#35925,#35926));
#6772=EDGE_LOOP('',(#35927,#35928,#35929,#35930));
#6773=EDGE_LOOP('',(#35931,#35932,#35933,#35934));
#6774=EDGE_LOOP('',(#35935,#35936,#35937,#35938));
#6775=EDGE_LOOP('',(#35939,#35940,#35941,#35942));
#6776=EDGE_LOOP('',(#35943,#35944));
#6777=EDGE_LOOP('',(#35945,#35946));
#6778=EDGE_LOOP('',(#35947,#35948,#35949,#35950,#35951,#35952,#35953,#35954,
#35955,#35956,#35957,#35958));
#6779=EDGE_LOOP('',(#35959,#35960,#35961,#35962));
#6780=EDGE_LOOP('',(#35963,#35964,#35965,#35966,#35967,#35968,#35969,#35970,
#35971,#35972));
#6781=EDGE_LOOP('',(#35973,#35974));
#8871=CIRCLE('',#44273,16.);
#8872=CIRCLE('',#44274,1.);
#8873=CIRCLE('',#44275,17.);
#8874=CIRCLE('',#44276,17.);
#8875=CIRCLE('',#44278,17.);
#8876=CIRCLE('',#44280,13.8);
#8877=CIRCLE('',#44282,18.);
#8878=CIRCLE('',#44283,1.);
#8879=CIRCLE('',#44284,19.);
#8880=CIRCLE('',#44285,19.);
#8881=CIRCLE('',#44287,19.);
#8882=CIRCLE('',#44290,23.548750780275);
#8883=CIRCLE('',#44291,1.);
#8884=CIRCLE('',#44292,24.5475031191528);
#8885=CIRCLE('',#44293,24.5475031191528);
#8886=CIRCLE('',#44295,25.);
#8887=CIRCLE('',#44298,40.7071067811865);
#8888=CIRCLE('',#44299,40.7071067811865);
#8889=CIRCLE('',#44300,1.);
#8890=CIRCLE('',#44301,41.);
#8891=CIRCLE('',#44302,41.);
#8892=CIRCLE('',#44304,41.);
#8893=CIRCLE('',#44305,41.);
#8894=CIRCLE('',#44307,39.);
#8895=CIRCLE('',#44308,39.);
#8896=CIRCLE('',#44309,39.);
#8897=CIRCLE('',#44310,39.);
#8898=CIRCLE('',#44311,39.);
#8899=CIRCLE('',#44312,39.);
#8900=CIRCLE('',#44313,39.);
#8901=CIRCLE('',#44315,1.);
#8902=CIRCLE('',#44316,40.7071067811866);
#8903=CIRCLE('',#44317,40.7071067811866);
#8904=CIRCLE('',#44319,40.6928932188135);
#8905=CIRCLE('',#44320,40.6928932188135);
#8906=CIRCLE('',#44322,0.999999999999999);
#8907=CIRCLE('',#44323,1.);
#8908=CIRCLE('',#44325,1.00000000000001);
#8909=CIRCLE('',#44326,15.5);
#8910=CIRCLE('',#44327,1.);
#8911=CIRCLE('',#44328,16.5);
#8912=CIRCLE('',#44330,1.);
#8913=CIRCLE('',#44332,1.);
#8914=CIRCLE('',#44333,1.);
#8915=CIRCLE('',#44335,1.);
#8916=CIRCLE('',#44337,18.);
#8917=CIRCLE('',#44338,18.);
#8918=CIRCLE('',#44340,19.);
#8919=CIRCLE('',#44341,1.00000000000001);
#8920=CIRCLE('',#44343,39.9857864376269);
#8921=CIRCLE('',#44344,19.);
#8922=CIRCLE('',#44345,16.5);
#8923=CIRCLE('',#44346,19.);
#8924=CIRCLE('',#44347,16.5);
#8925=CIRCLE('',#44349,18.);
#8926=CIRCLE('',#44350,1.);
#8927=CIRCLE('',#44352,18.);
#8928=CIRCLE('',#44354,1.);
#8929=CIRCLE('',#44355,1.);
#8930=CIRCLE('',#44357,1.);
#8931=CIRCLE('',#44359,15.5);
#8932=CIRCLE('',#44360,15.5);
#8933=CIRCLE('',#44362,1.00000000000001);
#8934=CIRCLE('',#44364,1.);
#8935=CIRCLE('',#44369,1.);
#8936=CIRCLE('',#44370,1.);
#8937=CIRCLE('',#44372,1.);
#8938=CIRCLE('',#44374,15.5);
#8939=CIRCLE('',#44375,1.);
#8940=CIRCLE('',#44377,15.5);
#8941=CIRCLE('',#44379,1.);
#8942=CIRCLE('',#44380,1.);
#8943=CIRCLE('',#44382,1.);
#8944=CIRCLE('',#44384,1.00000000000001);
#8945=CIRCLE('',#44385,18.);
#8946=CIRCLE('',#44387,1.);
#8947=CIRCLE('',#44389,18.);
#8948=CIRCLE('',#44391,1.);
#8949=CIRCLE('',#44393,38.);
#8950=CIRCLE('',#44394,39.);
#8951=CIRCLE('',#44395,39.);
#8952=CIRCLE('',#44398,39.);
#8953=CIRCLE('',#44400,38.);
#8954=CIRCLE('',#44403,38.);
#8955=CIRCLE('',#44407,39.);
#8956=CIRCLE('',#44408,38.);
#8957=CIRCLE('',#44412,39.);
#8958=CIRCLE('',#44414,39.);
#8959=CIRCLE('',#44416,38.);
#8960=CIRCLE('',#44420,39.);
#8961=CIRCLE('',#44421,38.);
#8962=CIRCLE('',#44425,0.999999999999999);
#8963=CIRCLE('',#44426,0.999999999999999);
#8964=CIRCLE('',#44427,0.999999999999999);
#8965=CIRCLE('',#44428,0.999999999999999);
#8966=CIRCLE('',#44429,0.999999999999999);
#8967=CIRCLE('',#44431,12.);
#8968=CIRCLE('',#44432,12.);
#8969=CIRCLE('',#44436,12.1);
#8970=CIRCLE('',#44437,1.);
#8971=CIRCLE('',#44438,12.1);
#8972=CIRCLE('',#44439,1.);
#8973=CIRCLE('',#44440,1.);
#8974=CIRCLE('',#44441,12.1);
#8975=CIRCLE('',#44442,1.);
#8976=CIRCLE('',#44443,0.999999999999999);
#8977=CIRCLE('',#44444,12.1);
#8978=CIRCLE('',#44445,0.999999999999999);
#8979=CIRCLE('',#44446,1.);
#8980=CIRCLE('',#44447,12.1);
#8981=CIRCLE('',#44448,1.);
#8982=CIRCLE('',#44449,1.);
#8983=CIRCLE('',#44450,12.1);
#8984=CIRCLE('',#44451,1.);
#8985=CIRCLE('',#44452,1.);
#8986=CIRCLE('',#44453,12.1);
#8987=CIRCLE('',#44454,1.);
#8988=CIRCLE('',#44455,1.);
#8989=CIRCLE('',#44456,12.1);
#8990=CIRCLE('',#44457,1.);
#8991=CIRCLE('',#44458,0.999999999999999);
#8992=CIRCLE('',#44459,12.1);
#8993=CIRCLE('',#44460,0.999999999999999);
#8994=CIRCLE('',#44461,1.);
#8995=CIRCLE('',#44462,12.1);
#8996=CIRCLE('',#44463,1.);
#8997=CIRCLE('',#44464,1.);
#8998=CIRCLE('',#44465,12.1);
#8999=CIRCLE('',#44466,1.);
#9000=CIRCLE('',#44467,1.);
#9001=CIRCLE('',#44468,12.1);
#9002=CIRCLE('',#44469,1.);
#9003=CIRCLE('',#44470,0.999999999999999);
#9004=CIRCLE('',#44471,12.1);
#9005=CIRCLE('',#44472,0.999999999999999);
#9006=CIRCLE('',#44473,0.999999999999999);
#9007=CIRCLE('',#44474,12.1);
#9008=CIRCLE('',#44475,0.999999999999999);
#9009=CIRCLE('',#44476,0.999999999999999);
#9010=CIRCLE('',#44477,12.1);
#9011=CIRCLE('',#44478,0.999999999999999);
#9012=CIRCLE('',#44479,1.);
#9013=CIRCLE('',#44480,12.1);
#9014=CIRCLE('',#44481,1.);
#9015=CIRCLE('',#44482,1.);
#9016=CIRCLE('',#44483,12.1);
#9017=CIRCLE('',#44484,1.);
#9018=CIRCLE('',#44485,1.);
#9019=CIRCLE('',#44486,12.1);
#9020=CIRCLE('',#44487,1.);
#9021=CIRCLE('',#44488,1.);
#9022=CIRCLE('',#44489,12.1);
#9023=CIRCLE('',#44490,1.);
#9024=CIRCLE('',#44491,1.);
#9025=CIRCLE('',#44492,12.1);
#9026=CIRCLE('',#44493,1.);
#9027=CIRCLE('',#44494,1.);
#9028=CIRCLE('',#44495,12.1);
#9029=CIRCLE('',#44496,1.);
#9030=CIRCLE('',#44497,1.);
#9031=CIRCLE('',#44498,12.1);
#9032=CIRCLE('',#44499,1.);
#9033=CIRCLE('',#44500,1.);
#9034=CIRCLE('',#44501,12.1);
#9035=CIRCLE('',#44502,1.);
#9036=CIRCLE('',#44503,1.);
#9037=CIRCLE('',#44504,12.1);
#9038=CIRCLE('',#44505,1.);
#9039=CIRCLE('',#44506,1.);
#9040=CIRCLE('',#44507,12.1);
#9041=CIRCLE('',#44508,1.);
#9042=CIRCLE('',#44509,1.);
#9043=CIRCLE('',#44510,12.1);
#9044=CIRCLE('',#44511,1.);
#9045=CIRCLE('',#44514,0.999999999999999);
#9046=CIRCLE('',#44517,1.);
#9047=CIRCLE('',#44518,1.);
#9048=CIRCLE('',#44519,1.);
#9049=CIRCLE('',#44521,12.);
#9050=CIRCLE('',#44522,12.);
#9051=CIRCLE('',#44527,1.);
#9052=CIRCLE('',#44528,1.);
#9053=CIRCLE('',#44529,1.);
#9054=CIRCLE('',#44531,12.);
#9055=CIRCLE('',#44532,12.);
#9056=CIRCLE('',#44537,0.999999999999999);
#9057=CIRCLE('',#44538,0.999999999999999);
#9058=CIRCLE('',#44539,0.999999999999999);
#9059=CIRCLE('',#44541,12.);
#9060=CIRCLE('',#44542,12.);
#9061=CIRCLE('',#44547,1.);
#9062=CIRCLE('',#44548,1.);
#9063=CIRCLE('',#44549,1.);
#9064=CIRCLE('',#44551,12.);
#9065=CIRCLE('',#44552,12.);
#9066=CIRCLE('',#44557,1.);
#9067=CIRCLE('',#44558,1.);
#9068=CIRCLE('',#44559,1.);
#9069=CIRCLE('',#44561,12.);
#9070=CIRCLE('',#44562,12.);
#9071=CIRCLE('',#44567,1.);
#9072=CIRCLE('',#44568,1.);
#9073=CIRCLE('',#44569,1.);
#9074=CIRCLE('',#44571,12.);
#9075=CIRCLE('',#44572,12.);
#9076=CIRCLE('',#44577,1.);
#9077=CIRCLE('',#44578,1.);
#9078=CIRCLE('',#44579,1.);
#9079=CIRCLE('',#44581,12.);
#9080=CIRCLE('',#44582,12.);
#9081=CIRCLE('',#44587,0.999999999999999);
#9082=CIRCLE('',#44588,0.999999999999999);
#9083=CIRCLE('',#44589,0.999999999999999);
#9084=CIRCLE('',#44591,12.);
#9085=CIRCLE('',#44592,12.);
#9086=CIRCLE('',#44597,1.);
#9087=CIRCLE('',#44598,1.);
#9088=CIRCLE('',#44599,1.);
#9089=CIRCLE('',#44601,12.);
#9090=CIRCLE('',#44602,12.);
#9091=CIRCLE('',#44607,1.);
#9092=CIRCLE('',#44608,1.);
#9093=CIRCLE('',#44609,1.);
#9094=CIRCLE('',#44611,12.);
#9095=CIRCLE('',#44612,12.);
#9096=CIRCLE('',#44617,1.);
#9097=CIRCLE('',#44618,1.);
#9098=CIRCLE('',#44619,1.);
#9099=CIRCLE('',#44621,12.);
#9100=CIRCLE('',#44622,12.);
#9101=CIRCLE('',#44627,0.999999999999999);
#9102=CIRCLE('',#44628,0.999999999999999);
#9103=CIRCLE('',#44629,0.999999999999999);
#9104=CIRCLE('',#44631,12.);
#9105=CIRCLE('',#44632,12.);
#9106=CIRCLE('',#44637,0.999999999999999);
#9107=CIRCLE('',#44638,0.999999999999999);
#9108=CIRCLE('',#44639,0.999999999999999);
#9109=CIRCLE('',#44641,12.);
#9110=CIRCLE('',#44642,12.);
#9111=CIRCLE('',#44647,0.999999999999999);
#9112=CIRCLE('',#44648,0.999999999999999);
#9113=CIRCLE('',#44649,0.999999999999999);
#9114=CIRCLE('',#44651,12.);
#9115=CIRCLE('',#44652,12.);
#9116=CIRCLE('',#44657,1.);
#9117=CIRCLE('',#44658,1.);
#9118=CIRCLE('',#44659,1.);
#9119=CIRCLE('',#44661,12.);
#9120=CIRCLE('',#44662,12.);
#9121=CIRCLE('',#44667,1.);
#9122=CIRCLE('',#44668,1.);
#9123=CIRCLE('',#44669,1.);
#9124=CIRCLE('',#44671,12.);
#9125=CIRCLE('',#44672,12.);
#9126=CIRCLE('',#44677,1.);
#9127=CIRCLE('',#44678,1.);
#9128=CIRCLE('',#44679,1.);
#9129=CIRCLE('',#44681,12.);
#9130=CIRCLE('',#44682,12.);
#9131=CIRCLE('',#44687,1.);
#9132=CIRCLE('',#44688,1.);
#9133=CIRCLE('',#44689,1.);
#9134=CIRCLE('',#44691,12.);
#9135=CIRCLE('',#44692,12.);
#9136=CIRCLE('',#44697,1.);
#9137=CIRCLE('',#44698,1.);
#9138=CIRCLE('',#44699,1.);
#9139=CIRCLE('',#44701,12.);
#9140=CIRCLE('',#44702,12.);
#9141=CIRCLE('',#44707,1.);
#9142=CIRCLE('',#44708,1.);
#9143=CIRCLE('',#44709,1.);
#9144=CIRCLE('',#44711,12.);
#9145=CIRCLE('',#44712,12.);
#9146=CIRCLE('',#44717,1.);
#9147=CIRCLE('',#44718,1.);
#9148=CIRCLE('',#44719,1.);
#9149=CIRCLE('',#44721,12.);
#9150=CIRCLE('',#44722,12.);
#9151=CIRCLE('',#44727,1.);
#9152=CIRCLE('',#44728,1.);
#9153=CIRCLE('',#44729,1.);
#9154=CIRCLE('',#44731,12.);
#9155=CIRCLE('',#44732,12.);
#9156=CIRCLE('',#44737,1.);
#9157=CIRCLE('',#44738,1.);
#9158=CIRCLE('',#44739,1.);
#9159=CIRCLE('',#44741,12.);
#9160=CIRCLE('',#44742,12.);
#9161=CIRCLE('',#44747,1.);
#9162=CIRCLE('',#44748,1.);
#9163=CIRCLE('',#44749,1.);
#9164=CIRCLE('',#44752,12.);
#9165=CIRCLE('',#44753,12.);
#9166=CIRCLE('',#44756,1.);
#9167=CIRCLE('',#44757,1.);
#9168=CIRCLE('',#44758,1.);
#9169=CIRCLE('',#44760,12.);
#9170=CIRCLE('',#44761,12.);
#9171=CIRCLE('',#44764,12.8);
#9172=CIRCLE('',#44765,1.);
#9173=CIRCLE('',#44766,13.8);
#9174=CIRCLE('',#44767,13.8);
#9175=CIRCLE('',#44768,12.8);
#9176=CIRCLE('',#44769,12.9);
#9177=CIRCLE('',#44771,12.9);
#9178=CIRCLE('',#44805,15.5);
#10234=B_SPLINE_CURVE_WITH_KNOTS('',3,(#87091,#87092,#87093,#87094,#87095,
#87096,#87097,#87098),.UNSPECIFIED.,.F.,.F.,(4,2,2,4),(-0.196195849903657,
-0.195599538890117,-0.152519692792675,-0.146000767490103),.UNSPECIFIED.);
#10235=B_SPLINE_CURVE_WITH_KNOTS('',3,(#87102,#87103,#87104,#87105,#87106,
#87107,#87108,#87109),.UNSPECIFIED.,.F.,.F.,(4,2,2,4),(-0.050053324667382,
-0.0434746559737304,0.,0.000601775969721257),.UNSPECIFIED.);
#10236=B_SPLINE_CURVE_WITH_KNOTS('',3,(#87113,#87114,#87115,#87116,#87117,
#87118,#87119,#87120),.UNSPECIFIED.,.F.,.F.,(4,2,2,4),(0.0388307934706334,
0.0718206189099945,0.202781150815222,0.333741682720449),.UNSPECIFIED.);
#10237=B_SPLINE_CURVE_WITH_KNOTS('',3,(#87124,#87125,#87126,#87127,#87128,
#87129,#87130,#87131),.UNSPECIFIED.,.F.,.F.,(4,2,2,4),(1.22818284528083,
1.35914337718606,1.49010390909129,1.52309373453065),.UNSPECIFIED.);
#10238=B_SPLINE_CURVE_WITH_KNOTS('',3,(#87135,#87136,#87137,#87138,#87139,
#87140,#87141,#87142),.UNSPECIFIED.,.F.,.F.,(4,2,2,4),(0.0388307934706321,
0.0718206189099869,0.202781150815209,0.333741682720432),.UNSPECIFIED.);
#10239=B_SPLINE_CURVE_WITH_KNOTS('',3,(#87145,#87146,#87147,#87148,#87149,
#87150,#87151,#87152),.UNSPECIFIED.,.F.,.F.,(4,2,2,4),(1.22818284528085,
1.35914337718607,1.4901039090913,1.52309373453065),.UNSPECIFIED.);
#10240=B_SPLINE_CURVE_WITH_KNOTS('',3,(#87155,#87156,#87157,#87158,#87159,
#87160,#87161,#87162),.UNSPECIFIED.,.F.,.F.,(4,2,2,4),(-0.196195849903479,
-0.195599538889944,-0.152519692792554,-0.146000767489991),.UNSPECIFIED.);
#10241=B_SPLINE_CURVE_WITH_KNOTS('',3,(#87164,#87165,#87166,#87167,#87168,
#87169,#87170,#87171),.UNSPECIFIED.,.F.,.F.,(4,2,2,4),(-0.0500533246673741,
-0.0434746559737304,0.,0.000601775969725807),.UNSPECIFIED.);
#10242=B_SPLINE_CURVE_WITH_KNOTS('',3,(#87223,#87224,#87225,#87226,#87227,
#87228,#87229,#87230),.UNSPECIFIED.,.F.,.F.,(4,2,2,4),(-0.451157298746012,
-0.450377434324763,-0.395988663028411,-0.389083946741513),.UNSPECIFIED.);
#10243=B_SPLINE_CURVE_WITH_KNOTS('',3,(#87232,#87233,#87234,#87235,#87236,
#87237,#87238,#87239),.UNSPECIFIED.,.F.,.F.,(4,2,2,4),(-1.52309373971353,
-1.4901039090913,-1.35914337718608,-1.22818284528086),.UNSPECIFIED.);
#10244=B_SPLINE_CURVE_WITH_KNOTS('',3,(#87243,#87244,#87245,#87246,#87247,
#87248,#87249,#87250),.UNSPECIFIED.,.F.,.F.,(4,2,2,4),(-0.333741682720433,
-0.202781150815209,-0.0718206189099861,-0.0388307882877552),
 .UNSPECIFIED.);
#10245=B_SPLINE_CURVE_WITH_KNOTS('',3,(#87251,#87252,#87253,#87254,#87255,
#87256),.UNSPECIFIED.,.F.,.F.,(4,2,4),(-0.0499943672376333,0.,0.000636386853239865),
 .UNSPECIFIED.);
#10246=B_SPLINE_CURVE_WITH_KNOTS('',3,(#87262,#87263,#87264,#87265,#87266,
#87267,#87268,#87269),.UNSPECIFIED.,.F.,.F.,(4,2,2,4),(-0.000636386853552818,
0.,0.0443824568631479,0.0500168601686062),.UNSPECIFIED.);
#10247=B_SPLINE_CURVE_WITH_KNOTS('',3,(#87274,#87275,#87276,#87277,#87278,
#87279),.UNSPECIFIED.,.F.,.F.,(4,2,4),(0.,0.0499385293981029,0.050574205481999),
 .UNSPECIFIED.);
#10248=B_SPLINE_CURVE_WITH_KNOTS('',3,(#87284,#87285,#87286,#87287,#87288,
#87289,#87290,#87291),.UNSPECIFIED.,.F.,.F.,(4,2,2,4),(-1.52309373971353,
-1.49010390909129,-1.35914337718606,-1.22818284528083),.UNSPECIFIED.);
#10249=B_SPLINE_CURVE_WITH_KNOTS('',3,(#87294,#87295,#87296,#87297,#87298,
#87299,#87300,#87301),.UNSPECIFIED.,.F.,.F.,(4,2,2,4),(-0.333741682720448,
-0.202781150815221,-0.0718206189099939,-0.0388307882877496),
 .UNSPECIFIED.);
#10250=B_SPLINE_CURVE_WITH_KNOTS('',3,(#87314,#87315,#87316,#87317,#87318,
#87319,#87320,#87321),.UNSPECIFIED.,.F.,.F.,(4,2,2,4),(-0.451157298521714,
-0.450377434100828,-0.39598866283428,-0.389083946550594),.UNSPECIFIED.);
#10251=B_SPLINE_CURVE_WITH_KNOTS('',3,(#87323,#87324,#87325,#87326,#87327,
#87328,#87329,#87330),.UNSPECIFIED.,.F.,.F.,(4,2,2,4),(-1.52309373971353,
-1.4901039090913,-1.35914337718608,-1.22818284528085),.UNSPECIFIED.);
#10252=B_SPLINE_CURVE_WITH_KNOTS('',3,(#87334,#87335,#87336,#87337,#87338,
#87339,#87340,#87341),.UNSPECIFIED.,.F.,.F.,(4,2,2,4),(-0.333741682720432,
-0.20278115081521,-0.071820618909987,-0.0388307882877565),.UNSPECIFIED.);
#10253=B_SPLINE_CURVE_WITH_KNOTS('',3,(#87342,#87343,#87344,#87345,#87346,
#87347),.UNSPECIFIED.,.F.,.F.,(4,2,4),(-0.0499943672375485,0.,0.00063638685309623),
 .UNSPECIFIED.);
#10254=B_SPLINE_CURVE_WITH_KNOTS('',3,(#87351,#87352,#87353,#87354,#87355,
#87356,#87357,#87358),.UNSPECIFIED.,.F.,.F.,(4,2,2,4),(-0.000636386853589343,
0.,0.0443824568628011,0.050016860168427),.UNSPECIFIED.);
#10255=B_SPLINE_CURVE_WITH_KNOTS('',3,(#87362,#87363,#87364,#87365,#87366,
#87367),.UNSPECIFIED.,.F.,.F.,(4,2,4),(0.,0.0499385293979143,0.0505742054816259),
 .UNSPECIFIED.);
#10256=B_SPLINE_CURVE_WITH_KNOTS('',3,(#87371,#87372,#87373,#87374,#87375,
#87376,#87377,#87378),.UNSPECIFIED.,.F.,.F.,(4,2,2,4),(-1.52309373971353,
-1.49010390909129,-1.35914337718606,-1.22818284528083),.UNSPECIFIED.);
#10257=B_SPLINE_CURVE_WITH_KNOTS('',3,(#87381,#87382,#87383,#87384,#87385,
#87386,#87387,#87388),.UNSPECIFIED.,.F.,.F.,(4,2,2,4),(-0.333741682720449,
-0.202781150815222,-0.0718206189099946,-0.0388307882877464),
 .UNSPECIFIED.);
#10258=B_SPLINE_CURVE_WITH_KNOTS('',3,(#87405,#87406,#87407,#87408,#87409,
#87410),.UNSPECIFIED.,.F.,.F.,(4,2,4),(0.177494794972093,0.193749996937672,
0.210005198903256),.UNSPECIFIED.);
#10259=B_SPLINE_CURVE_WITH_KNOTS('',3,(#87428,#87429,#87430,#87431),
 .UNSPECIFIED.,.F.,.F.,(4,4),(0.444630732493599,0.454287074896198),
 .UNSPECIFIED.);
#10260=B_SPLINE_CURVE_WITH_KNOTS('',3,(#87643,#87644,#87645,#87646,#87647,
#87648),.UNSPECIFIED.,.F.,.F.,(4,2,4),(-0.0472169084629657,-0.036873447077816,
0.),.UNSPECIFIED.);
#10261=B_SPLINE_CURVE_WITH_KNOTS('',3,(#87655,#87656,#87657,#87658,#87659,
#87660),.UNSPECIFIED.,.F.,.F.,(4,2,4),(0.523618879647139,0.539874081612722,
0.556129283578305),.UNSPECIFIED.);
#10262=B_SPLINE_CURVE_WITH_KNOTS('',3,(#87681,#87682,#87683,#87684,#87685,
#87686),.UNSPECIFIED.,.F.,.F.,(4,2,4),(0.523618879647142,0.539874081612723,
0.556129283578306),.UNSPECIFIED.);
#10263=B_SPLINE_CURVE_WITH_KNOTS('',3,(#87707,#87708,#87709,#87710,#87711,
#87712),.UNSPECIFIED.,.F.,.F.,(4,2,4),(0.523618879647138,0.539874081612722,
0.556129283578303),.UNSPECIFIED.);
#10264=B_SPLINE_CURVE_WITH_KNOTS('',3,(#87733,#87734,#87735,#87736,#87737,
#87738),.UNSPECIFIED.,.F.,.F.,(4,2,4),(0.523618879647139,0.539874081612722,
0.556129283578296),.UNSPECIFIED.);
#10265=B_SPLINE_CURVE_WITH_KNOTS('',3,(#87759,#87760,#87761,#87762,#87763,
#87764),.UNSPECIFIED.,.F.,.F.,(4,2,4),(0.523618879647139,0.539874081612722,
0.556129283578303),.UNSPECIFIED.);
#10266=B_SPLINE_CURVE_WITH_KNOTS('',3,(#87785,#87786,#87787,#87788,#87789,
#87790),.UNSPECIFIED.,.F.,.F.,(4,2,4),(0.52361887964714,0.539874081612723,
0.556129283578306),.UNSPECIFIED.);
#10267=B_SPLINE_CURVE_WITH_KNOTS('',3,(#87811,#87812,#87813,#87814,#87815,
#87816),.UNSPECIFIED.,.F.,.F.,(4,2,4),(0.523618879647139,0.539874081612722,
0.556129283578295),.UNSPECIFIED.);
#10268=B_SPLINE_CURVE_WITH_KNOTS('',3,(#87837,#87838,#87839,#87840,#87841,
#87842),.UNSPECIFIED.,.F.,.F.,(4,2,4),(0.52361887964713,0.539874081612714,
0.556129283578297),.UNSPECIFIED.);
#10269=B_SPLINE_CURVE_WITH_KNOTS('',3,(#87863,#87864,#87865,#87866,#87867,
#87868),.UNSPECIFIED.,.F.,.F.,(4,2,4),(0.523618879647139,0.539874081612722,
0.556129283578299),.UNSPECIFIED.);
#10270=B_SPLINE_CURVE_WITH_KNOTS('',3,(#87889,#87890,#87891,#87892,#87893,
#87894),.UNSPECIFIED.,.F.,.F.,(4,2,4),(0.523618879647144,0.539874081612722,
0.556129283578297),.UNSPECIFIED.);
#10271=B_SPLINE_CURVE_WITH_KNOTS('',3,(#87915,#87916,#87917,#87918,#87919,
#87920),.UNSPECIFIED.,.F.,.F.,(4,2,4),(0.523618879647139,0.539874081612722,
0.556129283578297),.UNSPECIFIED.);
#10272=B_SPLINE_CURVE_WITH_KNOTS('',3,(#87941,#87942,#87943,#87944,#87945,
#87946),.UNSPECIFIED.,.F.,.F.,(4,2,4),(0.52361887964713,0.539874081612714,
0.556129283578297),.UNSPECIFIED.);
#10273=B_SPLINE_CURVE_WITH_KNOTS('',3,(#87967,#87968,#87969,#87970,#87971,
#87972),.UNSPECIFIED.,.F.,.F.,(4,2,4),(0.523618879647139,0.539874081612722,
0.556129283578305),.UNSPECIFIED.);
#10274=B_SPLINE_CURVE_WITH_KNOTS('',3,(#87993,#87994,#87995,#87996,#87997,
#87998),.UNSPECIFIED.,.F.,.F.,(4,2,4),(0.523618879647138,0.539874081612714,
0.556129283578288),.UNSPECIFIED.);
#10275=B_SPLINE_CURVE_WITH_KNOTS('',3,(#88019,#88020,#88021,#88022,#88023,
#88024),.UNSPECIFIED.,.F.,.F.,(4,2,4),(0.523618879647142,0.539874081612723,
0.556129283578306),.UNSPECIFIED.);
#10276=B_SPLINE_CURVE_WITH_KNOTS('',3,(#88045,#88046,#88047,#88048,#88049,
#88050),.UNSPECIFIED.,.F.,.F.,(4,2,4),(0.523618879647139,0.539874081612722,
0.556129283578295),.UNSPECIFIED.);
#10277=B_SPLINE_CURVE_WITH_KNOTS('',3,(#88071,#88072,#88073,#88074,#88075,
#88076),.UNSPECIFIED.,.F.,.F.,(4,2,4),(0.523618879647139,0.539874081612722,
0.556129283578305),.UNSPECIFIED.);
#10278=B_SPLINE_CURVE_WITH_KNOTS('',3,(#88097,#88098,#88099,#88100,#88101,
#88102),.UNSPECIFIED.,.F.,.F.,(4,2,4),(0.523618879647139,0.539874081612722,
0.556129283578295),.UNSPECIFIED.);
#10279=B_SPLINE_CURVE_WITH_KNOTS('',3,(#88123,#88124,#88125,#88126,#88127,
#88128),.UNSPECIFIED.,.F.,.F.,(4,2,4),(0.52361887964714,0.539874081612713,
0.556129283578292),.UNSPECIFIED.);
#10280=B_SPLINE_CURVE_WITH_KNOTS('',3,(#88149,#88150,#88151,#88152,#88153,
#88154),.UNSPECIFIED.,.F.,.F.,(4,2,4),(0.523618879647135,0.539874081612718,
0.556129283578301),.UNSPECIFIED.);
#10281=B_SPLINE_CURVE_WITH_KNOTS('',3,(#88175,#88176,#88177,#88178,#88179,
#88180),.UNSPECIFIED.,.F.,.F.,(4,2,4),(0.523618879647139,0.539874081612722,
0.556129283578305),.UNSPECIFIED.);
#10282=B_SPLINE_CURVE_WITH_KNOTS('',3,(#88201,#88202,#88203,#88204,#88205,
#88206),.UNSPECIFIED.,.F.,.F.,(4,2,4),(0.523618879647148,0.539874081612722,
0.556129283578305),.UNSPECIFIED.);
#10283=B_SPLINE_CURVE_WITH_KNOTS('',3,(#88227,#88228,#88229,#88230,#88231,
#88232),.UNSPECIFIED.,.F.,.F.,(4,2,4),(0.523618879647147,0.539874081612722,
0.556129283578301),.UNSPECIFIED.);
#10284=B_SPLINE_CURVE_WITH_KNOTS('',3,(#88253,#88254,#88255,#88256,#88257,
#88258),.UNSPECIFIED.,.F.,.F.,(4,2,4),(0.523618879647122,0.539874081612714,
0.556129283578311),.UNSPECIFIED.);
#10285=B_SPLINE_CURVE_WITH_KNOTS('',3,(#88278,#88279,#88280,#88281,#88282,
#88283),.UNSPECIFIED.,.F.,.F.,(4,2,4),(0.523618879647139,0.539874081612723,
0.556129283578306),.UNSPECIFIED.);
#12346=LINE('',#86939,#14840);
#12347=LINE('',#86954,#14841);
#12348=LINE('',#86967,#14842);
#12349=LINE('',#86982,#14843);
#12350=LINE('',#87000,#14844);
#12351=LINE('',#87010,#14845);
#12352=LINE('',#87019,#14846);
#12353=LINE('',#87022,#14847);
#12354=LINE('',#87037,#14848);
#12355=LINE('',#87040,#14849);
#12356=LINE('',#87047,#14850);
#12357=LINE('',#87070,#14851);
#12358=LINE('',#87075,#14852);
#12359=LINE('',#87083,#14853);
#12360=LINE('',#87100,#14854);
#12361=LINE('',#87110,#14855);
#12362=LINE('',#87122,#14856);
#12363=LINE('',#87133,#14857);
#12364=LINE('',#87144,#14858);
#12365=LINE('',#87163,#14859);
#12366=LINE('',#87177,#14860);
#12367=LINE('',#87187,#14861);
#12368=LINE('',#87192,#14862);
#12369=LINE('',#87204,#14863);
#12370=LINE('',#87217,#14864);
#12371=LINE('',#87259,#14865);
#12372=LINE('',#87261,#14866);
#12373=LINE('',#87272,#14867);
#12374=LINE('',#87280,#14868);
#12375=LINE('',#87303,#14869);
#12376=LINE('',#87304,#14870);
#12377=LINE('',#87310,#14871);
#12378=LINE('',#87350,#14872);
#12379=LINE('',#87361,#14873);
#12380=LINE('',#87390,#14874);
#12381=LINE('',#87391,#14875);
#12382=LINE('',#87398,#14876);
#12383=LINE('',#87402,#14877);
#12384=LINE('',#87415,#14878);
#12385=LINE('',#87418,#14879);
#12386=LINE('',#87426,#14880);
#12387=LINE('',#87432,#14881);
#12388=LINE('',#87436,#14882);
#12389=LINE('',#87444,#14883);
#12390=LINE('',#87452,#14884);
#12391=LINE('',#87460,#14885);
#12392=LINE('',#87468,#14886);
#12393=LINE('',#87476,#14887);
#12394=LINE('',#87484,#14888);
#12395=LINE('',#87492,#14889);
#12396=LINE('',#87500,#14890);
#12397=LINE('',#87508,#14891);
#12398=LINE('',#87516,#14892);
#12399=LINE('',#87524,#14893);
#12400=LINE('',#87532,#14894);
#12401=LINE('',#87540,#14895);
#12402=LINE('',#87548,#14896);
#12403=LINE('',#87556,#14897);
#12404=LINE('',#87564,#14898);
#12405=LINE('',#87572,#14899);
#12406=LINE('',#87580,#14900);
#12407=LINE('',#87588,#14901);
#12408=LINE('',#87596,#14902);
#12409=LINE('',#87604,#14903);
#12410=LINE('',#87612,#14904);
#12411=LINE('',#87620,#14905);
#12412=LINE('',#87628,#14906);
#12413=LINE('',#87635,#14907);
#12414=LINE('',#87642,#14908);
#12415=LINE('',#87654,#14909);
#12416=LINE('',#87661,#14910);
#12417=LINE('',#87666,#14911);
#12418=LINE('',#87669,#14912);
#12419=LINE('',#87680,#14913);
#12420=LINE('',#87687,#14914);
#12421=LINE('',#87692,#14915);
#12422=LINE('',#87695,#14916);
#12423=LINE('',#87706,#14917);
#12424=LINE('',#87713,#14918);
#12425=LINE('',#87718,#14919);
#12426=LINE('',#87721,#14920);
#12427=LINE('',#87732,#14921);
#12428=LINE('',#87739,#14922);
#12429=LINE('',#87744,#14923);
#12430=LINE('',#87747,#14924);
#12431=LINE('',#87758,#14925);
#12432=LINE('',#87765,#14926);
#12433=LINE('',#87770,#14927);
#12434=LINE('',#87773,#14928);
#12435=LINE('',#87784,#14929);
#12436=LINE('',#87791,#14930);
#12437=LINE('',#87796,#14931);
#12438=LINE('',#87799,#14932);
#12439=LINE('',#87810,#14933);
#12440=LINE('',#87817,#14934);
#12441=LINE('',#87822,#14935);
#12442=LINE('',#87825,#14936);
#12443=LINE('',#87836,#14937);
#12444=LINE('',#87843,#14938);
#12445=LINE('',#87848,#14939);
#12446=LINE('',#87851,#14940);
#12447=LINE('',#87862,#14941);
#12448=LINE('',#87869,#14942);
#12449=LINE('',#87874,#14943);
#12450=LINE('',#87877,#14944);
#12451=LINE('',#87888,#14945);
#12452=LINE('',#87895,#14946);
#12453=LINE('',#87900,#14947);
#12454=LINE('',#87903,#14948);
#12455=LINE('',#87914,#14949);
#12456=LINE('',#87921,#14950);
#12457=LINE('',#87926,#14951);
#12458=LINE('',#87929,#14952);
#12459=LINE('',#87940,#14953);
#12460=LINE('',#87947,#14954);
#12461=LINE('',#87952,#14955);
#12462=LINE('',#87955,#14956);
#12463=LINE('',#87966,#14957);
#12464=LINE('',#87973,#14958);
#12465=LINE('',#87978,#14959);
#12466=LINE('',#87981,#14960);
#12467=LINE('',#87992,#14961);
#12468=LINE('',#87999,#14962);
#12469=LINE('',#88004,#14963);
#12470=LINE('',#88007,#14964);
#12471=LINE('',#88018,#14965);
#12472=LINE('',#88025,#14966);
#12473=LINE('',#88030,#14967);
#12474=LINE('',#88033,#14968);
#12475=LINE('',#88044,#14969);
#12476=LINE('',#88051,#14970);
#12477=LINE('',#88056,#14971);
#12478=LINE('',#88059,#14972);
#12479=LINE('',#88070,#14973);
#12480=LINE('',#88077,#14974);
#12481=LINE('',#88082,#14975);
#12482=LINE('',#88085,#14976);
#12483=LINE('',#88096,#14977);
#12484=LINE('',#88103,#14978);
#12485=LINE('',#88108,#14979);
#12486=LINE('',#88111,#14980);
#12487=LINE('',#88122,#14981);
#12488=LINE('',#88129,#14982);
#12489=LINE('',#88134,#14983);
#12490=LINE('',#88137,#14984);
#12491=LINE('',#88148,#14985);
#12492=LINE('',#88155,#14986);
#12493=LINE('',#88160,#14987);
#12494=LINE('',#88163,#14988);
#12495=LINE('',#88174,#14989);
#12496=LINE('',#88181,#14990);
#12497=LINE('',#88186,#14991);
#12498=LINE('',#88189,#14992);
#12499=LINE('',#88200,#14993);
#12500=LINE('',#88207,#14994);
#12501=LINE('',#88212,#14995);
#12502=LINE('',#88215,#14996);
#12503=LINE('',#88226,#14997);
#12504=LINE('',#88233,#14998);
#12505=LINE('',#88238,#14999);
#12506=LINE('',#88241,#15000);
#12507=LINE('',#88252,#15001);
#12508=LINE('',#88259,#15002);
#12509=LINE('',#88264,#15003);
#12510=LINE('',#88267,#15004);
#12511=LINE('',#88277,#15005);
#12512=LINE('',#88284,#15006);
#12513=LINE('',#88289,#15007);
#12514=LINE('',#88292,#15008);
#12515=LINE('',#88309,#15009);
#12516=LINE('',#88310,#15010);
#12517=LINE('',#88311,#15011);
#12518=LINE('',#88312,#15012);
#12519=LINE('',#88313,#15013);
#12520=LINE('',#88314,#15014);
#12521=LINE('',#88315,#15015);
#12522=LINE('',#88316,#15016);
#12523=LINE('',#88317,#15017);
#12524=LINE('',#88318,#15018);
#12525=LINE('',#88319,#15019);
#12526=LINE('',#88320,#15020);
#12527=LINE('',#88321,#15021);
#12528=LINE('',#88322,#15022);
#12529=LINE('',#88323,#15023);
#12530=LINE('',#88324,#15024);
#12531=LINE('',#88325,#15025);
#12532=LINE('',#88326,#15026);
#12533=LINE('',#88327,#15027);
#12534=LINE('',#88328,#15028);
#12535=LINE('',#88329,#15029);
#12536=LINE('',#88330,#15030);
#12537=LINE('',#88331,#15031);
#12538=LINE('',#88332,#15032);
#12539=LINE('',#88333,#15033);
#12540=LINE('',#88334,#15034);
#12541=LINE('',#88336,#15035);
#12542=LINE('',#88372,#15036);
#14840=VECTOR('',#54740,17.);
#14841=VECTOR('',#54759,19.);
#14842=VECTOR('',#54776,24.75);
#14843=VECTOR('',#54795,41.);
#14844=VECTOR('',#54814,40.);
#14845=VECTOR('',#54827,40.7);
#14846=VECTOR('',#54836,10.);
#14847=VECTOR('',#54839,10.);
#14848=VECTOR('',#54858,10.);
#14849=VECTOR('',#54861,10.);
#14850=VECTOR('',#54870,10.);
#14851=VECTOR('',#54901,10.);
#14852=VECTOR('',#54906,10.);
#14853=VECTOR('',#54917,10.);
#14854=VECTOR('',#54930,10.);
#14855=VECTOR('',#54931,10.);
#14856=VECTOR('',#54934,10.);
#14857=VECTOR('',#54935,10.);
#14858=VECTOR('',#54936,10.);
#14859=VECTOR('',#54939,10.);
#14860=VECTOR('',#54946,10.);
#14861=VECTOR('',#54961,10.);
#14862=VECTOR('',#54966,10.);
#14863=VECTOR('',#54985,10.);
#14864=VECTOR('',#55006,10.);
#14865=VECTOR('',#55019,10.);
#14866=VECTOR('',#55020,10.);
#14867=VECTOR('',#55023,10.);
#14868=VECTOR('',#55024,10.);
#14869=VECTOR('',#55033,10.);
#14870=VECTOR('',#55034,10.);
#14871=VECTOR('',#55043,10.);
#14872=VECTOR('',#55052,10.);
#14873=VECTOR('',#55055,10.);
#14874=VECTOR('',#55064,10.);
#14875=VECTOR('',#55065,10.);
#14876=VECTOR('',#55072,10.);
#14877=VECTOR('',#55075,10.);
#14878=VECTOR('',#55080,10.);
#14879=VECTOR('',#55083,10.);
#14880=VECTOR('',#55094,10.);
#14881=VECTOR('',#55095,10.);
#14882=VECTOR('',#55100,10.);
#14883=VECTOR('',#55107,10.);
#14884=VECTOR('',#55114,10.);
#14885=VECTOR('',#55121,10.);
#14886=VECTOR('',#55128,10.);
#14887=VECTOR('',#55135,10.);
#14888=VECTOR('',#55142,10.);
#14889=VECTOR('',#55149,10.);
#14890=VECTOR('',#55156,10.);
#14891=VECTOR('',#55163,10.);
#14892=VECTOR('',#55170,10.);
#14893=VECTOR('',#55177,10.);
#14894=VECTOR('',#55184,10.);
#14895=VECTOR('',#55191,10.);
#14896=VECTOR('',#55198,10.);
#14897=VECTOR('',#55205,10.);
#14898=VECTOR('',#55212,10.);
#14899=VECTOR('',#55219,10.);
#14900=VECTOR('',#55226,10.);
#14901=VECTOR('',#55233,10.);
#14902=VECTOR('',#55240,10.);
#14903=VECTOR('',#55247,10.);
#14904=VECTOR('',#55254,10.);
#14905=VECTOR('',#55261,10.);
#14906=VECTOR('',#55268,10.);
#14907=VECTOR('',#55275,10.);
#14908=VECTOR('',#55282,1.);
#14909=VECTOR('',#55289,10.);
#14910=VECTOR('',#55290,10.);
#14911=VECTOR('',#55293,10.);
#14912=VECTOR('',#55296,10.);
#14913=VECTOR('',#55313,10.);
#14914=VECTOR('',#55314,10.);
#14915=VECTOR('',#55317,10.);
#14916=VECTOR('',#55320,10.);
#14917=VECTOR('',#55337,10.);
#14918=VECTOR('',#55338,10.);
#14919=VECTOR('',#55341,10.);
#14920=VECTOR('',#55344,10.);
#14921=VECTOR('',#55361,10.);
#14922=VECTOR('',#55362,10.);
#14923=VECTOR('',#55365,10.);
#14924=VECTOR('',#55368,10.);
#14925=VECTOR('',#55385,10.);
#14926=VECTOR('',#55386,10.);
#14927=VECTOR('',#55389,10.);
#14928=VECTOR('',#55392,10.);
#14929=VECTOR('',#55409,10.);
#14930=VECTOR('',#55410,10.);
#14931=VECTOR('',#55413,10.);
#14932=VECTOR('',#55416,10.);
#14933=VECTOR('',#55433,10.);
#14934=VECTOR('',#55434,10.);
#14935=VECTOR('',#55437,10.);
#14936=VECTOR('',#55440,10.);
#14937=VECTOR('',#55457,10.);
#14938=VECTOR('',#55458,10.);
#14939=VECTOR('',#55461,10.);
#14940=VECTOR('',#55464,10.);
#14941=VECTOR('',#55481,10.);
#14942=VECTOR('',#55482,10.);
#14943=VECTOR('',#55485,10.);
#14944=VECTOR('',#55488,10.);
#14945=VECTOR('',#55505,10.);
#14946=VECTOR('',#55506,10.);
#14947=VECTOR('',#55509,10.);
#14948=VECTOR('',#55512,10.);
#14949=VECTOR('',#55529,10.);
#14950=VECTOR('',#55530,10.);
#14951=VECTOR('',#55533,10.);
#14952=VECTOR('',#55536,10.);
#14953=VECTOR('',#55553,10.);
#14954=VECTOR('',#55554,10.);
#14955=VECTOR('',#55557,10.);
#14956=VECTOR('',#55560,10.);
#14957=VECTOR('',#55577,10.);
#14958=VECTOR('',#55578,10.);
#14959=VECTOR('',#55581,10.);
#14960=VECTOR('',#55584,10.);
#14961=VECTOR('',#55601,10.);
#14962=VECTOR('',#55602,10.);
#14963=VECTOR('',#55605,10.);
#14964=VECTOR('',#55608,10.);
#14965=VECTOR('',#55625,10.);
#14966=VECTOR('',#55626,10.);
#14967=VECTOR('',#55629,10.);
#14968=VECTOR('',#55632,10.);
#14969=VECTOR('',#55649,10.);
#14970=VECTOR('',#55650,10.);
#14971=VECTOR('',#55653,10.);
#14972=VECTOR('',#55656,10.);
#14973=VECTOR('',#55673,10.);
#14974=VECTOR('',#55674,10.);
#14975=VECTOR('',#55677,10.);
#14976=VECTOR('',#55680,10.);
#14977=VECTOR('',#55697,10.);
#14978=VECTOR('',#55698,10.);
#14979=VECTOR('',#55701,10.);
#14980=VECTOR('',#55704,10.);
#14981=VECTOR('',#55721,10.);
#14982=VECTOR('',#55722,10.);
#14983=VECTOR('',#55725,10.);
#14984=VECTOR('',#55728,10.);
#14985=VECTOR('',#55745,10.);
#14986=VECTOR('',#55746,10.);
#14987=VECTOR('',#55749,10.);
#14988=VECTOR('',#55752,10.);
#14989=VECTOR('',#55769,10.);
#14990=VECTOR('',#55770,10.);
#14991=VECTOR('',#55773,10.);
#14992=VECTOR('',#55776,10.);
#14993=VECTOR('',#55793,10.);
#14994=VECTOR('',#55794,10.);
#14995=VECTOR('',#55797,10.);
#14996=VECTOR('',#55800,10.);
#14997=VECTOR('',#55817,10.);
#14998=VECTOR('',#55818,10.);
#14999=VECTOR('',#55821,10.);
#15000=VECTOR('',#55824,10.);
#15001=VECTOR('',#55841,10.);
#15002=VECTOR('',#55842,10.);
#15003=VECTOR('',#55845,10.);
#15004=VECTOR('',#55848,10.);
#15005=VECTOR('',#55863,10.);
#15006=VECTOR('',#55864,10.);
#15007=VECTOR('',#55867,10.);
#15008=VECTOR('',#55870,10.);
#15009=VECTOR('',#55897,10.);
#15010=VECTOR('',#55898,10.);
#15011=VECTOR('',#55899,10.);
#15012=VECTOR('',#55900,10.);
#15013=VECTOR('',#55901,10.);
#15014=VECTOR('',#55902,10.);
#15015=VECTOR('',#55903,10.);
#15016=VECTOR('',#55904,10.);
#15017=VECTOR('',#55905,10.);
#15018=VECTOR('',#55906,10.);
#15019=VECTOR('',#55907,10.);
#15020=VECTOR('',#55908,10.);
#15021=VECTOR('',#55909,10.);
#15022=VECTOR('',#55910,10.);
#15023=VECTOR('',#55911,10.);
#15024=VECTOR('',#55912,10.);
#15025=VECTOR('',#55913,10.);
#15026=VECTOR('',#55914,10.);
#15027=VECTOR('',#55915,10.);
#15028=VECTOR('',#55916,10.);
#15029=VECTOR('',#55917,10.);
#15030=VECTOR('',#55918,10.);
#15031=VECTOR('',#55919,10.);
#15032=VECTOR('',#55920,10.);
#15033=VECTOR('',#55921,10.);
#15034=VECTOR('',#55922,10.);
#15035=VECTOR('',#55925,13.8);
#15036=VECTOR('',#55996,32.);
#18302=VERTEX_POINT('',#86930);
#18303=VERTEX_POINT('',#86932);
#18304=VERTEX_POINT('',#86934);
#18305=VERTEX_POINT('',#86938);
#18306=VERTEX_POINT('',#86942);
#18307=VERTEX_POINT('',#86945);
#18308=VERTEX_POINT('',#86947);
#18309=VERTEX_POINT('',#86949);
#18310=VERTEX_POINT('',#86953);
#18311=VERTEX_POINT('',#86958);
#18312=VERTEX_POINT('',#86960);
#18313=VERTEX_POINT('',#86962);
#18314=VERTEX_POINT('',#86966);
#18315=VERTEX_POINT('',#86971);
#18316=VERTEX_POINT('',#86972);
#18317=VERTEX_POINT('',#86975);
#18318=VERTEX_POINT('',#86977);
#18319=VERTEX_POINT('',#86981);
#18320=VERTEX_POINT('',#86983);
#18321=VERTEX_POINT('',#86987);
#18322=VERTEX_POINT('',#86988);
#18323=VERTEX_POINT('',#86990);
#18324=VERTEX_POINT('',#86992);
#18325=VERTEX_POINT('',#86994);
#18326=VERTEX_POINT('',#86996);
#18327=VERTEX_POINT('',#86998);
#18328=VERTEX_POINT('',#87003);
#18329=VERTEX_POINT('',#87005);
#18330=VERTEX_POINT('',#87009);
#18331=VERTEX_POINT('',#87011);
#18332=VERTEX_POINT('',#87015);
#18333=VERTEX_POINT('',#87016);
#18334=VERTEX_POINT('',#87018);
#18335=VERTEX_POINT('',#87020);
#18336=VERTEX_POINT('',#87024);
#18337=VERTEX_POINT('',#87026);
#18338=VERTEX_POINT('',#87028);
#18339=VERTEX_POINT('',#87034);
#18340=VERTEX_POINT('',#87036);
#18341=VERTEX_POINT('',#87038);
#18342=VERTEX_POINT('',#87044);
#18343=VERTEX_POINT('',#87046);
#18344=VERTEX_POINT('',#87050);
#18345=VERTEX_POINT('',#87054);
#18346=VERTEX_POINT('',#87056);
#18347=VERTEX_POINT('',#87058);
#18348=VERTEX_POINT('',#87060);
#18349=VERTEX_POINT('',#87064);
#18350=VERTEX_POINT('',#87068);
#18351=VERTEX_POINT('',#87072);
#18352=VERTEX_POINT('',#87074);
#18353=VERTEX_POINT('',#87080);
#18354=VERTEX_POINT('',#87082);
#18355=VERTEX_POINT('',#87090);
#18356=VERTEX_POINT('',#87099);
#18357=VERTEX_POINT('',#87101);
#18358=VERTEX_POINT('',#87112);
#18359=VERTEX_POINT('',#87121);
#18360=VERTEX_POINT('',#87123);
#18361=VERTEX_POINT('',#87132);
#18362=VERTEX_POINT('',#87134);
#18363=VERTEX_POINT('',#87143);
#18364=VERTEX_POINT('',#87154);
#18365=VERTEX_POINT('',#87173);
#18366=VERTEX_POINT('',#87175);
#18367=VERTEX_POINT('',#87181);
#18368=VERTEX_POINT('',#87185);
#18369=VERTEX_POINT('',#87189);
#18370=VERTEX_POINT('',#87191);
#18371=VERTEX_POINT('',#87197);
#18372=VERTEX_POINT('',#87203);
#18373=VERTEX_POINT('',#87210);
#18374=VERTEX_POINT('',#87215);
#18375=VERTEX_POINT('',#87222);
#18376=VERTEX_POINT('',#87231);
#18377=VERTEX_POINT('',#87240);
#18378=VERTEX_POINT('',#87242);
#18379=VERTEX_POINT('',#87258);
#18380=VERTEX_POINT('',#87260);
#18381=VERTEX_POINT('',#87271);
#18382=VERTEX_POINT('',#87273);
#18383=VERTEX_POINT('',#87283);
#18384=VERTEX_POINT('',#87292);
#18385=VERTEX_POINT('',#87309);
#18386=VERTEX_POINT('',#87313);
#18387=VERTEX_POINT('',#87322);
#18388=VERTEX_POINT('',#87331);
#18389=VERTEX_POINT('',#87333);
#18390=VERTEX_POINT('',#87349);
#18391=VERTEX_POINT('',#87360);
#18392=VERTEX_POINT('',#87370);
#18393=VERTEX_POINT('',#87379);
#18394=VERTEX_POINT('',#87394);
#18395=VERTEX_POINT('',#87395);
#18396=VERTEX_POINT('',#87397);
#18397=VERTEX_POINT('',#87399);
#18398=VERTEX_POINT('',#87401);
#18399=VERTEX_POINT('',#87403);
#18400=VERTEX_POINT('',#87411);
#18401=VERTEX_POINT('',#87412);
#18402=VERTEX_POINT('',#87414);
#18403=VERTEX_POINT('',#87416);
#18404=VERTEX_POINT('',#87424);
#18405=VERTEX_POINT('',#87425);
#18406=VERTEX_POINT('',#87427);
#18407=VERTEX_POINT('',#87435);
#18408=VERTEX_POINT('',#87437);
#18409=VERTEX_POINT('',#87439);
#18410=VERTEX_POINT('',#87441);
#18411=VERTEX_POINT('',#87443);
#18412=VERTEX_POINT('',#87445);
#18413=VERTEX_POINT('',#87447);
#18414=VERTEX_POINT('',#87449);
#18415=VERTEX_POINT('',#87451);
#18416=VERTEX_POINT('',#87453);
#18417=VERTEX_POINT('',#87455);
#18418=VERTEX_POINT('',#87457);
#18419=VERTEX_POINT('',#87459);
#18420=VERTEX_POINT('',#87461);
#18421=VERTEX_POINT('',#87463);
#18422=VERTEX_POINT('',#87465);
#18423=VERTEX_POINT('',#87467);
#18424=VERTEX_POINT('',#87469);
#18425=VERTEX_POINT('',#87471);
#18426=VERTEX_POINT('',#87473);
#18427=VERTEX_POINT('',#87475);
#18428=VERTEX_POINT('',#87477);
#18429=VERTEX_POINT('',#87479);
#18430=VERTEX_POINT('',#87481);
#18431=VERTEX_POINT('',#87483);
#18432=VERTEX_POINT('',#87485);
#18433=VERTEX_POINT('',#87487);
#18434=VERTEX_POINT('',#87489);
#18435=VERTEX_POINT('',#87491);
#18436=VERTEX_POINT('',#87493);
#18437=VERTEX_POINT('',#87495);
#18438=VERTEX_POINT('',#87497);
#18439=VERTEX_POINT('',#87499);
#18440=VERTEX_POINT('',#87501);
#18441=VERTEX_POINT('',#87503);
#18442=VERTEX_POINT('',#87505);
#18443=VERTEX_POINT('',#87507);
#18444=VERTEX_POINT('',#87509);
#18445=VERTEX_POINT('',#87511);
#18446=VERTEX_POINT('',#87513);
#18447=VERTEX_POINT('',#87515);
#18448=VERTEX_POINT('',#87517);
#18449=VERTEX_POINT('',#87519);
#18450=VERTEX_POINT('',#87521);
#18451=VERTEX_POINT('',#87523);
#18452=VERTEX_POINT('',#87525);
#18453=VERTEX_POINT('',#87527);
#18454=VERTEX_POINT('',#87529);
#18455=VERTEX_POINT('',#87531);
#18456=VERTEX_POINT('',#87533);
#18457=VERTEX_POINT('',#87535);
#18458=VERTEX_POINT('',#87537);
#18459=VERTEX_POINT('',#87539);
#18460=VERTEX_POINT('',#87541);
#18461=VERTEX_POINT('',#87543);
#18462=VERTEX_POINT('',#87545);
#18463=VERTEX_POINT('',#87547);
#18464=VERTEX_POINT('',#87549);
#18465=VERTEX_POINT('',#87551);
#18466=VERTEX_POINT('',#87553);
#18467=VERTEX_POINT('',#87555);
#18468=VERTEX_POINT('',#87557);
#18469=VERTEX_POINT('',#87559);
#18470=VERTEX_POINT('',#87561);
#18471=VERTEX_POINT('',#87563);
#18472=VERTEX_POINT('',#87565);
#18473=VERTEX_POINT('',#87567);
#18474=VERTEX_POINT('',#87569);
#18475=VERTEX_POINT('',#87571);
#18476=VERTEX_POINT('',#87573);
#18477=VERTEX_POINT('',#87575);
#18478=VERTEX_POINT('',#87577);
#18479=VERTEX_POINT('',#87579);
#18480=VERTEX_POINT('',#87581);
#18481=VERTEX_POINT('',#87583);
#18482=VERTEX_POINT('',#87585);
#18483=VERTEX_POINT('',#87587);
#18484=VERTEX_POINT('',#87589);
#18485=VERTEX_POINT('',#87591);
#18486=VERTEX_POINT('',#87593);
#18487=VERTEX_POINT('',#87595);
#18488=VERTEX_POINT('',#87597);
#18489=VERTEX_POINT('',#87599);
#18490=VERTEX_POINT('',#87601);
#18491=VERTEX_POINT('',#87603);
#18492=VERTEX_POINT('',#87605);
#18493=VERTEX_POINT('',#87607);
#18494=VERTEX_POINT('',#87609);
#18495=VERTEX_POINT('',#87611);
#18496=VERTEX_POINT('',#87613);
#18497=VERTEX_POINT('',#87615);
#18498=VERTEX_POINT('',#87617);
#18499=VERTEX_POINT('',#87619);
#18500=VERTEX_POINT('',#87621);
#18501=VERTEX_POINT('',#87623);
#18502=VERTEX_POINT('',#87625);
#18503=VERTEX_POINT('',#87627);
#18504=VERTEX_POINT('',#87629);
#18505=VERTEX_POINT('',#87631);
#18506=VERTEX_POINT('',#87633);
#18507=VERTEX_POINT('',#87638);
#18508=VERTEX_POINT('',#87639);
#18509=VERTEX_POINT('',#87641);
#18510=VERTEX_POINT('',#87651);
#18511=VERTEX_POINT('',#87652);
#18512=VERTEX_POINT('',#87662);
#18513=VERTEX_POINT('',#87663);
#18514=VERTEX_POINT('',#87665);
#18515=VERTEX_POINT('',#87667);
#18516=VERTEX_POINT('',#87677);
#18517=VERTEX_POINT('',#87678);
#18518=VERTEX_POINT('',#87688);
#18519=VERTEX_POINT('',#87689);
#18520=VERTEX_POINT('',#87691);
#18521=VERTEX_POINT('',#87693);
#18522=VERTEX_POINT('',#87703);
#18523=VERTEX_POINT('',#87704);
#18524=VERTEX_POINT('',#87714);
#18525=VERTEX_POINT('',#87715);
#18526=VERTEX_POINT('',#87717);
#18527=VERTEX_POINT('',#87719);
#18528=VERTEX_POINT('',#87729);
#18529=VERTEX_POINT('',#87730);
#18530=VERTEX_POINT('',#87740);
#18531=VERTEX_POINT('',#87741);
#18532=VERTEX_POINT('',#87743);
#18533=VERTEX_POINT('',#87745);
#18534=VERTEX_POINT('',#87755);
#18535=VERTEX_POINT('',#87756);
#18536=VERTEX_POINT('',#87766);
#18537=VERTEX_POINT('',#87767);
#18538=VERTEX_POINT('',#87769);
#18539=VERTEX_POINT('',#87771);
#18540=VERTEX_POINT('',#87781);
#18541=VERTEX_POINT('',#87782);
#18542=VERTEX_POINT('',#87792);
#18543=VERTEX_POINT('',#87793);
#18544=VERTEX_POINT('',#87795);
#18545=VERTEX_POINT('',#87797);
#18546=VERTEX_POINT('',#87807);
#18547=VERTEX_POINT('',#87808);
#18548=VERTEX_POINT('',#87818);
#18549=VERTEX_POINT('',#87819);
#18550=VERTEX_POINT('',#87821);
#18551=VERTEX_POINT('',#87823);
#18552=VERTEX_POINT('',#87833);
#18553=VERTEX_POINT('',#87834);
#18554=VERTEX_POINT('',#87844);
#18555=VERTEX_POINT('',#87845);
#18556=VERTEX_POINT('',#87847);
#18557=VERTEX_POINT('',#87849);
#18558=VERTEX_POINT('',#87859);
#18559=VERTEX_POINT('',#87860);
#18560=VERTEX_POINT('',#87870);
#18561=VERTEX_POINT('',#87871);
#18562=VERTEX_POINT('',#87873);
#18563=VERTEX_POINT('',#87875);
#18564=VERTEX_POINT('',#87885);
#18565=VERTEX_POINT('',#87886);
#18566=VERTEX_POINT('',#87896);
#18567=VERTEX_POINT('',#87897);
#18568=VERTEX_POINT('',#87899);
#18569=VERTEX_POINT('',#87901);
#18570=VERTEX_POINT('',#87911);
#18571=VERTEX_POINT('',#87912);
#18572=VERTEX_POINT('',#87922);
#18573=VERTEX_POINT('',#87923);
#18574=VERTEX_POINT('',#87925);
#18575=VERTEX_POINT('',#87927);
#18576=VERTEX_POINT('',#87937);
#18577=VERTEX_POINT('',#87938);
#18578=VERTEX_POINT('',#87948);
#18579=VERTEX_POINT('',#87949);
#18580=VERTEX_POINT('',#87951);
#18581=VERTEX_POINT('',#87953);
#18582=VERTEX_POINT('',#87963);
#18583=VERTEX_POINT('',#87964);
#18584=VERTEX_POINT('',#87974);
#18585=VERTEX_POINT('',#87975);
#18586=VERTEX_POINT('',#87977);
#18587=VERTEX_POINT('',#87979);
#18588=VERTEX_POINT('',#87989);
#18589=VERTEX_POINT('',#87990);
#18590=VERTEX_POINT('',#88000);
#18591=VERTEX_POINT('',#88001);
#18592=VERTEX_POINT('',#88003);
#18593=VERTEX_POINT('',#88005);
#18594=VERTEX_POINT('',#88015);
#18595=VERTEX_POINT('',#88016);
#18596=VERTEX_POINT('',#88026);
#18597=VERTEX_POINT('',#88027);
#18598=VERTEX_POINT('',#88029);
#18599=VERTEX_POINT('',#88031);
#18600=VERTEX_POINT('',#88041);
#18601=VERTEX_POINT('',#88042);
#18602=VERTEX_POINT('',#88052);
#18603=VERTEX_POINT('',#88053);
#18604=VERTEX_POINT('',#88055);
#18605=VERTEX_POINT('',#88057);
#18606=VERTEX_POINT('',#88067);
#18607=VERTEX_POINT('',#88068);
#18608=VERTEX_POINT('',#88078);
#18609=VERTEX_POINT('',#88079);
#18610=VERTEX_POINT('',#88081);
#18611=VERTEX_POINT('',#88083);
#18612=VERTEX_POINT('',#88093);
#18613=VERTEX_POINT('',#88094);
#18614=VERTEX_POINT('',#88104);
#18615=VERTEX_POINT('',#88105);
#18616=VERTEX_POINT('',#88107);
#18617=VERTEX_POINT('',#88109);
#18618=VERTEX_POINT('',#88119);
#18619=VERTEX_POINT('',#88120);
#18620=VERTEX_POINT('',#88130);
#18621=VERTEX_POINT('',#88131);
#18622=VERTEX_POINT('',#88133);
#18623=VERTEX_POINT('',#88135);
#18624=VERTEX_POINT('',#88145);
#18625=VERTEX_POINT('',#88146);
#18626=VERTEX_POINT('',#88156);
#18627=VERTEX_POINT('',#88157);
#18628=VERTEX_POINT('',#88159);
#18629=VERTEX_POINT('',#88161);
#18630=VERTEX_POINT('',#88171);
#18631=VERTEX_POINT('',#88172);
#18632=VERTEX_POINT('',#88182);
#18633=VERTEX_POINT('',#88183);
#18634=VERTEX_POINT('',#88185);
#18635=VERTEX_POINT('',#88187);
#18636=VERTEX_POINT('',#88197);
#18637=VERTEX_POINT('',#88198);
#18638=VERTEX_POINT('',#88208);
#18639=VERTEX_POINT('',#88209);
#18640=VERTEX_POINT('',#88211);
#18641=VERTEX_POINT('',#88213);
#18642=VERTEX_POINT('',#88223);
#18643=VERTEX_POINT('',#88224);
#18644=VERTEX_POINT('',#88234);
#18645=VERTEX_POINT('',#88235);
#18646=VERTEX_POINT('',#88237);
#18647=VERTEX_POINT('',#88239);
#18648=VERTEX_POINT('',#88249);
#18649=VERTEX_POINT('',#88250);
#18650=VERTEX_POINT('',#88260);
#18651=VERTEX_POINT('',#88261);
#18652=VERTEX_POINT('',#88263);
#18653=VERTEX_POINT('',#88265);
#18654=VERTEX_POINT('',#88274);
#18655=VERTEX_POINT('',#88275);
#18656=VERTEX_POINT('',#88285);
#18657=VERTEX_POINT('',#88286);
#18658=VERTEX_POINT('',#88288);
#18659=VERTEX_POINT('',#88290);
#18660=VERTEX_POINT('',#88298);
#18661=VERTEX_POINT('',#88300);
#18662=VERTEX_POINT('',#88302);
#23942=EDGE_CURVE('',#18302,#18302,#8871,.T.);
#23943=EDGE_CURVE('',#18302,#18303,#8872,.T.);
#23944=EDGE_CURVE('',#18303,#18304,#8873,.T.);
#23945=EDGE_CURVE('',#18304,#18303,#8874,.T.);
#23946=EDGE_CURVE('',#18304,#18305,#12346,.T.);
#23947=EDGE_CURVE('',#18305,#18305,#8875,.T.);
#23948=EDGE_CURVE('',#18306,#18306,#8876,.T.);
#23949=EDGE_CURVE('',#18307,#18307,#8877,.T.);
#23950=EDGE_CURVE('',#18307,#18308,#8878,.T.);
#23951=EDGE_CURVE('',#18308,#18309,#8879,.T.);
#23952=EDGE_CURVE('',#18309,#18308,#8880,.T.);
#23953=EDGE_CURVE('',#18309,#18310,#12347,.T.);
#23954=EDGE_CURVE('',#18310,#18310,#8881,.T.);
#23955=EDGE_CURVE('',#18311,#18311,#8882,.T.);
#23956=EDGE_CURVE('',#18311,#18312,#8883,.T.);
#23957=EDGE_CURVE('',#18312,#18313,#8884,.T.);
#23958=EDGE_CURVE('',#18313,#18312,#8885,.T.);
#23959=EDGE_CURVE('',#18313,#18314,#12348,.T.);
#23960=EDGE_CURVE('',#18314,#18314,#8886,.T.);
#23961=EDGE_CURVE('',#18315,#18316,#8887,.T.);
#23962=EDGE_CURVE('',#18316,#18315,#8888,.T.);
#23963=EDGE_CURVE('',#18315,#18317,#8889,.T.);
#23964=EDGE_CURVE('',#18317,#18318,#8890,.T.);
#23965=EDGE_CURVE('',#18318,#18317,#8891,.T.);
#23966=EDGE_CURVE('',#18318,#18319,#12349,.T.);
#23967=EDGE_CURVE('',#18320,#18319,#8892,.T.);
#23968=EDGE_CURVE('',#18319,#18320,#8893,.T.);
#23969=EDGE_CURVE('',#18321,#18322,#8894,.T.);
#23970=EDGE_CURVE('',#18323,#18321,#8895,.T.);
#23971=EDGE_CURVE('',#18324,#18323,#8896,.T.);
#23972=EDGE_CURVE('',#18325,#18324,#8897,.T.);
#23973=EDGE_CURVE('',#18326,#18325,#8898,.T.);
#23974=EDGE_CURVE('',#18327,#18326,#8899,.T.);
#23975=EDGE_CURVE('',#18327,#18316,#12350,.T.);
#23976=EDGE_CURVE('',#18322,#18327,#8900,.T.);
#23977=EDGE_CURVE('',#18320,#18328,#8901,.T.);
#23978=EDGE_CURVE('',#18328,#18329,#8902,.T.);
#23979=EDGE_CURVE('',#18329,#18328,#8903,.T.);
#23980=EDGE_CURVE('',#18329,#18330,#12351,.T.);
#23981=EDGE_CURVE('',#18331,#18330,#8904,.T.);
#23982=EDGE_CURVE('',#18330,#18331,#8905,.T.);
#23983=EDGE_CURVE('',#18332,#18333,#8906,.T.);
#23984=EDGE_CURVE('',#18333,#18334,#12352,.T.);
#23985=EDGE_CURVE('',#18334,#18335,#8907,.F.);
#23986=EDGE_CURVE('',#18335,#18332,#12353,.T.);
#23987=EDGE_CURVE('',#18336,#18332,#8908,.T.);
#23988=EDGE_CURVE('',#18332,#18337,#8909,.T.);
#23989=EDGE_CURVE('',#18337,#18338,#8910,.T.);
#23990=EDGE_CURVE('',#18338,#18336,#8911,.T.);
#23991=EDGE_CURVE('',#18336,#18333,#8912,.T.);
#23992=EDGE_CURVE('',#18339,#18337,#8913,.T.);
#23993=EDGE_CURVE('',#18337,#18340,#12354,.T.);
#23994=EDGE_CURVE('',#18340,#18341,#8914,.F.);
#23995=EDGE_CURVE('',#18341,#18339,#12355,.T.);
#23996=EDGE_CURVE('',#18339,#18338,#8915,.T.);
#23997=EDGE_CURVE('',#18342,#18333,#8916,.T.);
#23998=EDGE_CURVE('',#18343,#18342,#12356,.T.);
#23999=EDGE_CURVE('',#18343,#18334,#8917,.T.);
#24000=EDGE_CURVE('',#18336,#18344,#8918,.T.);
#24001=EDGE_CURVE('',#18344,#18342,#8919,.T.);
#24002=EDGE_CURVE('',#18345,#18345,#8920,.T.);
#24003=EDGE_CURVE('',#18346,#18338,#8921,.T.);
#24004=EDGE_CURVE('',#18347,#18346,#8922,.T.);
#24005=EDGE_CURVE('',#18348,#18347,#8923,.T.);
#24006=EDGE_CURVE('',#18344,#18348,#8924,.T.);
#24007=EDGE_CURVE('',#18339,#18349,#8925,.T.);
#24008=EDGE_CURVE('',#18349,#18346,#8926,.T.);
#24009=EDGE_CURVE('',#18341,#18350,#8927,.T.);
#24010=EDGE_CURVE('',#18349,#18350,#12357,.T.);
#24011=EDGE_CURVE('',#18342,#18351,#8928,.T.);
#24012=EDGE_CURVE('',#18351,#18352,#12358,.T.);
#24013=EDGE_CURVE('',#18352,#18343,#8929,.F.);
#24014=EDGE_CURVE('',#18344,#18351,#8930,.T.);
#24015=EDGE_CURVE('',#18353,#18351,#8931,.T.);
#24016=EDGE_CURVE('',#18354,#18353,#12359,.T.);
#24017=EDGE_CURVE('',#18354,#18352,#8932,.T.);
#24018=EDGE_CURVE('',#18348,#18353,#8933,.T.);
#24019=EDGE_CURVE('',#18331,#18345,#8934,.T.);
#24020=EDGE_CURVE('',#18326,#18355,#10234,.T.);
#24021=EDGE_CURVE('',#18326,#18356,#12360,.T.);
#24022=EDGE_CURVE('',#18356,#18357,#10235,.F.);
#24023=EDGE_CURVE('',#18357,#18355,#12361,.T.);
#24024=EDGE_CURVE('',#18358,#18357,#10236,.F.);
#24025=EDGE_CURVE('',#18358,#18359,#12362,.T.);
#24026=EDGE_CURVE('',#18360,#18359,#10237,.F.);
#24027=EDGE_CURVE('',#18361,#18360,#12363,.T.);
#24028=EDGE_CURVE('',#18362,#18361,#10238,.F.);
#24029=EDGE_CURVE('',#18363,#18362,#12364,.T.);
#24030=EDGE_CURVE('',#18355,#18363,#10239,.F.);
#24031=EDGE_CURVE('',#18364,#18360,#10240,.T.);
#24032=EDGE_CURVE('',#18364,#18322,#12365,.T.);
#24033=EDGE_CURVE('',#18322,#18361,#10241,.F.);
#24034=EDGE_CURVE('',#18365,#18349,#8935,.T.);
#24035=EDGE_CURVE('',#18350,#18366,#8936,.F.);
#24036=EDGE_CURVE('',#18366,#18365,#12366,.T.);
#24037=EDGE_CURVE('',#18365,#18346,#8937,.T.);
#24038=EDGE_CURVE('',#18365,#18367,#8938,.T.);
#24039=EDGE_CURVE('',#18367,#18347,#8939,.T.);
#24040=EDGE_CURVE('',#18366,#18368,#8940,.T.);
#24041=EDGE_CURVE('',#18367,#18368,#12367,.T.);
#24042=EDGE_CURVE('',#18353,#18369,#8941,.T.);
#24043=EDGE_CURVE('',#18369,#18370,#12368,.T.);
#24044=EDGE_CURVE('',#18370,#18354,#8942,.F.);
#24045=EDGE_CURVE('',#18348,#18369,#8943,.T.);
#24046=EDGE_CURVE('',#18347,#18371,#8944,.T.);
#24047=EDGE_CURVE('',#18371,#18369,#8945,.T.);
#24048=EDGE_CURVE('',#18367,#18371,#8946,.T.);
#24049=EDGE_CURVE('',#18372,#18371,#12369,.T.);
#24050=EDGE_CURVE('',#18372,#18370,#8947,.T.);
#24051=EDGE_CURVE('',#18368,#18372,#8948,.F.);
#24052=EDGE_CURVE('',#18359,#18358,#8949,.T.);
#24053=EDGE_CURVE('',#18373,#18356,#8950,.T.);
#24054=EDGE_CURVE('',#18364,#18373,#8951,.T.);
#24055=EDGE_CURVE('',#18374,#18364,#8952,.T.);
#24056=EDGE_CURVE('',#18321,#18374,#12370,.T.);
#24057=EDGE_CURVE('',#18363,#18362,#8953,.T.);
#24058=EDGE_CURVE('',#18324,#18375,#10242,.T.);
#24059=EDGE_CURVE('',#18375,#18376,#10243,.T.);
#24060=EDGE_CURVE('',#18376,#18377,#8954,.T.);
#24061=EDGE_CURVE('',#18377,#18378,#10244,.T.);
#24062=EDGE_CURVE('',#18378,#18325,#10245,.T.);
#24063=EDGE_CURVE('',#18379,#18375,#12371,.T.);
#24064=EDGE_CURVE('',#18324,#18380,#12372,.T.);
#24065=EDGE_CURVE('',#18380,#18379,#10246,.T.);
#24066=EDGE_CURVE('',#18378,#18381,#12373,.T.);
#24067=EDGE_CURVE('',#18381,#18382,#10247,.T.);
#24068=EDGE_CURVE('',#18382,#18325,#12374,.T.);
#24069=EDGE_CURVE('',#18382,#18380,#8955,.T.);
#24070=EDGE_CURVE('',#18381,#18383,#10248,.T.);
#24071=EDGE_CURVE('',#18383,#18384,#8956,.T.);
#24072=EDGE_CURVE('',#18384,#18379,#10249,.T.);
#24073=EDGE_CURVE('',#18376,#18377,#12375,.T.);
#24074=EDGE_CURVE('',#18384,#18383,#12376,.T.);
#24075=EDGE_CURVE('',#18356,#18382,#8957,.T.);
#24076=EDGE_CURVE('',#18385,#18323,#12377,.T.);
#24077=EDGE_CURVE('',#18380,#18385,#8958,.T.);
#24078=EDGE_CURVE('',#18321,#18386,#10250,.T.);
#24079=EDGE_CURVE('',#18386,#18387,#10251,.T.);
#24080=EDGE_CURVE('',#18387,#18388,#8959,.T.);
#24081=EDGE_CURVE('',#18388,#18389,#10252,.T.);
#24082=EDGE_CURVE('',#18389,#18323,#10253,.T.);
#24083=EDGE_CURVE('',#18390,#18386,#12378,.T.);
#24084=EDGE_CURVE('',#18374,#18390,#10254,.T.);
#24085=EDGE_CURVE('',#18389,#18391,#12379,.T.);
#24086=EDGE_CURVE('',#18391,#18385,#10255,.T.);
#24087=EDGE_CURVE('',#18385,#18374,#8960,.T.);
#24088=EDGE_CURVE('',#18391,#18392,#10256,.T.);
#24089=EDGE_CURVE('',#18392,#18393,#8961,.T.);
#24090=EDGE_CURVE('',#18393,#18390,#10257,.T.);
#24091=EDGE_CURVE('',#18387,#18388,#12380,.T.);
#24092=EDGE_CURVE('',#18393,#18392,#12381,.T.);
#24093=EDGE_CURVE('',#18394,#18395,#8962,.T.);
#24094=EDGE_CURVE('',#18396,#18395,#12382,.T.);
#24095=EDGE_CURVE('',#18396,#18397,#8963,.F.);
#24096=EDGE_CURVE('',#18397,#18398,#12383,.T.);
#24097=EDGE_CURVE('',#18398,#18399,#8964,.T.);
#24098=EDGE_CURVE('',#18399,#18394,#10258,.T.);
#24099=EDGE_CURVE('',#18400,#18401,#8965,.T.);
#24100=EDGE_CURVE('',#18401,#18402,#12384,.T.);
#24101=EDGE_CURVE('',#18402,#18403,#8966,.T.);
#24102=EDGE_CURVE('',#18403,#18400,#12385,.T.);
#24103=EDGE_CURVE('',#18401,#18400,#8967,.T.);
#24104=EDGE_CURVE('',#18402,#18403,#8968,.T.);
#24105=EDGE_CURVE('',#18404,#18405,#12386,.T.);
#24106=EDGE_CURVE('',#18404,#18406,#10259,.T.);
#24107=EDGE_CURVE('',#18406,#18405,#12387,.F.);
#24108=EDGE_CURVE('',#18394,#18399,#8969,.T.);
#24109=EDGE_CURVE('',#18398,#18407,#12388,.T.);
#24110=EDGE_CURVE('',#18408,#18407,#8970,.T.);
#24111=EDGE_CURVE('',#18408,#18409,#8971,.T.);
#24112=EDGE_CURVE('',#18410,#18409,#8972,.T.);
#24113=EDGE_CURVE('',#18410,#18411,#12389,.T.);
#24114=EDGE_CURVE('',#18412,#18411,#8973,.T.);
#24115=EDGE_CURVE('',#18412,#18413,#8974,.T.);
#24116=EDGE_CURVE('',#18414,#18413,#8975,.T.);
#24117=EDGE_CURVE('',#18414,#18415,#12390,.T.);
#24118=EDGE_CURVE('',#18416,#18415,#8976,.T.);
#24119=EDGE_CURVE('',#18416,#18417,#8977,.T.);
#24120=EDGE_CURVE('',#18418,#18417,#8978,.T.);
#24121=EDGE_CURVE('',#18418,#18419,#12391,.T.);
#24122=EDGE_CURVE('',#18420,#18419,#8979,.T.);
#24123=EDGE_CURVE('',#18420,#18421,#8980,.T.);
#24124=EDGE_CURVE('',#18422,#18421,#8981,.T.);
#24125=EDGE_CURVE('',#18422,#18423,#12392,.T.);
#24126=EDGE_CURVE('',#18424,#18423,#8982,.T.);
#24127=EDGE_CURVE('',#18424,#18425,#8983,.T.);
#24128=EDGE_CURVE('',#18426,#18425,#8984,.T.);
#24129=EDGE_CURVE('',#18426,#18427,#12393,.T.);
#24130=EDGE_CURVE('',#18428,#18427,#8985,.T.);
#24131=EDGE_CURVE('',#18428,#18429,#8986,.T.);
#24132=EDGE_CURVE('',#18430,#18429,#8987,.T.);
#24133=EDGE_CURVE('',#18430,#18431,#12394,.T.);
#24134=EDGE_CURVE('',#18432,#18431,#8988,.T.);
#24135=EDGE_CURVE('',#18432,#18433,#8989,.T.);
#24136=EDGE_CURVE('',#18434,#18433,#8990,.T.);
#24137=EDGE_CURVE('',#18434,#18435,#12395,.T.);
#24138=EDGE_CURVE('',#18436,#18435,#8991,.T.);
#24139=EDGE_CURVE('',#18436,#18437,#8992,.T.);
#24140=EDGE_CURVE('',#18438,#18437,#8993,.T.);
#24141=EDGE_CURVE('',#18438,#18439,#12396,.T.);
#24142=EDGE_CURVE('',#18440,#18439,#8994,.T.);
#24143=EDGE_CURVE('',#18440,#18441,#8995,.T.);
#24144=EDGE_CURVE('',#18442,#18441,#8996,.T.);
#24145=EDGE_CURVE('',#18442,#18443,#12397,.T.);
#24146=EDGE_CURVE('',#18444,#18443,#8997,.T.);
#24147=EDGE_CURVE('',#18444,#18445,#8998,.T.);
#24148=EDGE_CURVE('',#18446,#18445,#8999,.T.);
#24149=EDGE_CURVE('',#18446,#18447,#12398,.T.);
#24150=EDGE_CURVE('',#18448,#18447,#9000,.T.);
#24151=EDGE_CURVE('',#18448,#18449,#9001,.T.);
#24152=EDGE_CURVE('',#18450,#18449,#9002,.T.);
#24153=EDGE_CURVE('',#18450,#18451,#12399,.T.);
#24154=EDGE_CURVE('',#18452,#18451,#9003,.T.);
#24155=EDGE_CURVE('',#18452,#18453,#9004,.T.);
#24156=EDGE_CURVE('',#18454,#18453,#9005,.T.);
#24157=EDGE_CURVE('',#18454,#18455,#12400,.T.);
#24158=EDGE_CURVE('',#18456,#18455,#9006,.T.);
#24159=EDGE_CURVE('',#18456,#18457,#9007,.T.);
#24160=EDGE_CURVE('',#18458,#18457,#9008,.T.);
#24161=EDGE_CURVE('',#18458,#18459,#12401,.T.);
#24162=EDGE_CURVE('',#18460,#18459,#9009,.T.);
#24163=EDGE_CURVE('',#18460,#18461,#9010,.T.);
#24164=EDGE_CURVE('',#18462,#18461,#9011,.T.);
#24165=EDGE_CURVE('',#18462,#18463,#12402,.T.);
#24166=EDGE_CURVE('',#18464,#18463,#9012,.T.);
#24167=EDGE_CURVE('',#18464,#18465,#9013,.T.);
#24168=EDGE_CURVE('',#18466,#18465,#9014,.T.);
#24169=EDGE_CURVE('',#18466,#18467,#12403,.T.);
#24170=EDGE_CURVE('',#18468,#18467,#9015,.T.);
#24171=EDGE_CURVE('',#18468,#18469,#9016,.T.);
#24172=EDGE_CURVE('',#18470,#18469,#9017,.T.);
#24173=EDGE_CURVE('',#18470,#18471,#12404,.T.);
#24174=EDGE_CURVE('',#18472,#18471,#9018,.T.);
#24175=EDGE_CURVE('',#18472,#18473,#9019,.T.);
#24176=EDGE_CURVE('',#18474,#18473,#9020,.T.);
#24177=EDGE_CURVE('',#18474,#18475,#12405,.T.);
#24178=EDGE_CURVE('',#18476,#18475,#9021,.T.);
#24179=EDGE_CURVE('',#18476,#18477,#9022,.T.);
#24180=EDGE_CURVE('',#18478,#18477,#9023,.T.);
#24181=EDGE_CURVE('',#18478,#18479,#12406,.T.);
#24182=EDGE_CURVE('',#18480,#18479,#9024,.T.);
#24183=EDGE_CURVE('',#18480,#18481,#9025,.T.);
#24184=EDGE_CURVE('',#18482,#18481,#9026,.T.);
#24185=EDGE_CURVE('',#18482,#18483,#12407,.T.);
#24186=EDGE_CURVE('',#18484,#18483,#9027,.T.);
#24187=EDGE_CURVE('',#18484,#18485,#9028,.T.);
#24188=EDGE_CURVE('',#18486,#18485,#9029,.T.);
#24189=EDGE_CURVE('',#18486,#18487,#12408,.T.);
#24190=EDGE_CURVE('',#18488,#18487,#9030,.T.);
#24191=EDGE_CURVE('',#18488,#18489,#9031,.T.);
#24192=EDGE_CURVE('',#18490,#18489,#9032,.T.);
#24193=EDGE_CURVE('',#18490,#18491,#12409,.T.);
#24194=EDGE_CURVE('',#18492,#18491,#9033,.T.);
#24195=EDGE_CURVE('',#18492,#18493,#9034,.T.);
#24196=EDGE_CURVE('',#18494,#18493,#9035,.T.);
#24197=EDGE_CURVE('',#18494,#18495,#12410,.T.);
#24198=EDGE_CURVE('',#18496,#18495,#9036,.T.);
#24199=EDGE_CURVE('',#18496,#18497,#9037,.T.);
#24200=EDGE_CURVE('',#18498,#18497,#9038,.T.);
#24201=EDGE_CURVE('',#18498,#18499,#12411,.T.);
#24202=EDGE_CURVE('',#18500,#18499,#9039,.T.);
#24203=EDGE_CURVE('',#18500,#18501,#9040,.T.);
#24204=EDGE_CURVE('',#18502,#18501,#9041,.T.);
#24205=EDGE_CURVE('',#18502,#18503,#12412,.T.);
#24206=EDGE_CURVE('',#18504,#18503,#9042,.T.);
#24207=EDGE_CURVE('',#18504,#18505,#9043,.T.);
#24208=EDGE_CURVE('',#18506,#18505,#9044,.T.);
#24209=EDGE_CURVE('',#18506,#18395,#12413,.T.);
#24210=EDGE_CURVE('',#18507,#18508,#9045,.T.);
#24211=EDGE_CURVE('',#18507,#18509,#12414,.T.);
#24212=EDGE_CURVE('',#18509,#18508,#10260,.F.);
#24213=EDGE_CURVE('',#18510,#18511,#9046,.T.);
#24214=EDGE_CURVE('',#18510,#18410,#12415,.T.);
#24215=EDGE_CURVE('',#18409,#18408,#10261,.T.);
#24216=EDGE_CURVE('',#18511,#18407,#12416,.T.);
#24217=EDGE_CURVE('',#18512,#18513,#9047,.T.);
#24218=EDGE_CURVE('',#18513,#18514,#12417,.T.);
#24219=EDGE_CURVE('',#18514,#18515,#9048,.T.);
#24220=EDGE_CURVE('',#18515,#18512,#12418,.T.);
#24221=EDGE_CURVE('',#18513,#18512,#9049,.T.);
#24222=EDGE_CURVE('',#18514,#18515,#9050,.T.);
#24223=EDGE_CURVE('',#18516,#18517,#9051,.T.);
#24224=EDGE_CURVE('',#18516,#18414,#12419,.T.);
#24225=EDGE_CURVE('',#18413,#18412,#10262,.T.);
#24226=EDGE_CURVE('',#18517,#18411,#12420,.T.);
#24227=EDGE_CURVE('',#18518,#18519,#9052,.T.);
#24228=EDGE_CURVE('',#18519,#18520,#12421,.T.);
#24229=EDGE_CURVE('',#18520,#18521,#9053,.T.);
#24230=EDGE_CURVE('',#18521,#18518,#12422,.T.);
#24231=EDGE_CURVE('',#18519,#18518,#9054,.T.);
#24232=EDGE_CURVE('',#18520,#18521,#9055,.T.);
#24233=EDGE_CURVE('',#18522,#18523,#9056,.T.);
#24234=EDGE_CURVE('',#18522,#18418,#12423,.T.);
#24235=EDGE_CURVE('',#18417,#18416,#10263,.T.);
#24236=EDGE_CURVE('',#18523,#18415,#12424,.T.);
#24237=EDGE_CURVE('',#18524,#18525,#9057,.T.);
#24238=EDGE_CURVE('',#18525,#18526,#12425,.T.);
#24239=EDGE_CURVE('',#18526,#18527,#9058,.T.);
#24240=EDGE_CURVE('',#18527,#18524,#12426,.T.);
#24241=EDGE_CURVE('',#18525,#18524,#9059,.T.);
#24242=EDGE_CURVE('',#18526,#18527,#9060,.T.);
#24243=EDGE_CURVE('',#18528,#18529,#9061,.T.);
#24244=EDGE_CURVE('',#18528,#18422,#12427,.T.);
#24245=EDGE_CURVE('',#18421,#18420,#10264,.T.);
#24246=EDGE_CURVE('',#18529,#18419,#12428,.T.);
#24247=EDGE_CURVE('',#18530,#18531,#9062,.T.);
#24248=EDGE_CURVE('',#18531,#18532,#12429,.T.);
#24249=EDGE_CURVE('',#18532,#18533,#9063,.T.);
#24250=EDGE_CURVE('',#18533,#18530,#12430,.T.);
#24251=EDGE_CURVE('',#18531,#18530,#9064,.T.);
#24252=EDGE_CURVE('',#18532,#18533,#9065,.T.);
#24253=EDGE_CURVE('',#18534,#18535,#9066,.T.);
#24254=EDGE_CURVE('',#18534,#18426,#12431,.T.);
#24255=EDGE_CURVE('',#18425,#18424,#10265,.T.);
#24256=EDGE_CURVE('',#18535,#18423,#12432,.T.);
#24257=EDGE_CURVE('',#18536,#18537,#9067,.T.);
#24258=EDGE_CURVE('',#18537,#18538,#12433,.T.);
#24259=EDGE_CURVE('',#18538,#18539,#9068,.T.);
#24260=EDGE_CURVE('',#18539,#18536,#12434,.T.);
#24261=EDGE_CURVE('',#18537,#18536,#9069,.T.);
#24262=EDGE_CURVE('',#18538,#18539,#9070,.T.);
#24263=EDGE_CURVE('',#18540,#18541,#9071,.T.);
#24264=EDGE_CURVE('',#18540,#18430,#12435,.T.);
#24265=EDGE_CURVE('',#18429,#18428,#10266,.T.);
#24266=EDGE_CURVE('',#18541,#18427,#12436,.T.);
#24267=EDGE_CURVE('',#18542,#18543,#9072,.T.);
#24268=EDGE_CURVE('',#18543,#18544,#12437,.T.);
#24269=EDGE_CURVE('',#18544,#18545,#9073,.T.);
#24270=EDGE_CURVE('',#18545,#18542,#12438,.T.);
#24271=EDGE_CURVE('',#18543,#18542,#9074,.T.);
#24272=EDGE_CURVE('',#18544,#18545,#9075,.T.);
#24273=EDGE_CURVE('',#18546,#18547,#9076,.T.);
#24274=EDGE_CURVE('',#18546,#18434,#12439,.T.);
#24275=EDGE_CURVE('',#18433,#18432,#10267,.T.);
#24276=EDGE_CURVE('',#18547,#18431,#12440,.T.);
#24277=EDGE_CURVE('',#18548,#18549,#9077,.T.);
#24278=EDGE_CURVE('',#18549,#18550,#12441,.T.);
#24279=EDGE_CURVE('',#18550,#18551,#9078,.T.);
#24280=EDGE_CURVE('',#18551,#18548,#12442,.T.);
#24281=EDGE_CURVE('',#18549,#18548,#9079,.T.);
#24282=EDGE_CURVE('',#18550,#18551,#9080,.T.);
#24283=EDGE_CURVE('',#18552,#18553,#9081,.T.);
#24284=EDGE_CURVE('',#18552,#18438,#12443,.T.);
#24285=EDGE_CURVE('',#18437,#18436,#10268,.T.);
#24286=EDGE_CURVE('',#18553,#18435,#12444,.T.);
#24287=EDGE_CURVE('',#18554,#18555,#9082,.T.);
#24288=EDGE_CURVE('',#18555,#18556,#12445,.T.);
#24289=EDGE_CURVE('',#18556,#18557,#9083,.T.);
#24290=EDGE_CURVE('',#18557,#18554,#12446,.T.);
#24291=EDGE_CURVE('',#18555,#18554,#9084,.T.);
#24292=EDGE_CURVE('',#18556,#18557,#9085,.T.);
#24293=EDGE_CURVE('',#18558,#18559,#9086,.T.);
#24294=EDGE_CURVE('',#18558,#18442,#12447,.T.);
#24295=EDGE_CURVE('',#18441,#18440,#10269,.T.);
#24296=EDGE_CURVE('',#18559,#18439,#12448,.T.);
#24297=EDGE_CURVE('',#18560,#18561,#9087,.T.);
#24298=EDGE_CURVE('',#18561,#18562,#12449,.T.);
#24299=EDGE_CURVE('',#18562,#18563,#9088,.T.);
#24300=EDGE_CURVE('',#18563,#18560,#12450,.T.);
#24301=EDGE_CURVE('',#18561,#18560,#9089,.T.);
#24302=EDGE_CURVE('',#18562,#18563,#9090,.T.);
#24303=EDGE_CURVE('',#18564,#18565,#9091,.T.);
#24304=EDGE_CURVE('',#18564,#18446,#12451,.T.);
#24305=EDGE_CURVE('',#18445,#18444,#10270,.T.);
#24306=EDGE_CURVE('',#18565,#18443,#12452,.T.);
#24307=EDGE_CURVE('',#18566,#18567,#9092,.T.);
#24308=EDGE_CURVE('',#18567,#18568,#12453,.T.);
#24309=EDGE_CURVE('',#18568,#18569,#9093,.T.);
#24310=EDGE_CURVE('',#18569,#18566,#12454,.T.);
#24311=EDGE_CURVE('',#18567,#18566,#9094,.T.);
#24312=EDGE_CURVE('',#18568,#18569,#9095,.T.);
#24313=EDGE_CURVE('',#18570,#18571,#9096,.T.);
#24314=EDGE_CURVE('',#18570,#18450,#12455,.T.);
#24315=EDGE_CURVE('',#18449,#18448,#10271,.T.);
#24316=EDGE_CURVE('',#18571,#18447,#12456,.T.);
#24317=EDGE_CURVE('',#18572,#18573,#9097,.T.);
#24318=EDGE_CURVE('',#18573,#18574,#12457,.T.);
#24319=EDGE_CURVE('',#18574,#18575,#9098,.T.);
#24320=EDGE_CURVE('',#18575,#18572,#12458,.T.);
#24321=EDGE_CURVE('',#18573,#18572,#9099,.T.);
#24322=EDGE_CURVE('',#18574,#18575,#9100,.T.);
#24323=EDGE_CURVE('',#18576,#18577,#9101,.T.);
#24324=EDGE_CURVE('',#18576,#18454,#12459,.T.);
#24325=EDGE_CURVE('',#18453,#18452,#10272,.T.);
#24326=EDGE_CURVE('',#18577,#18451,#12460,.T.);
#24327=EDGE_CURVE('',#18578,#18579,#9102,.T.);
#24328=EDGE_CURVE('',#18579,#18580,#12461,.T.);
#24329=EDGE_CURVE('',#18580,#18581,#9103,.T.);
#24330=EDGE_CURVE('',#18581,#18578,#12462,.T.);
#24331=EDGE_CURVE('',#18579,#18578,#9104,.T.);
#24332=EDGE_CURVE('',#18580,#18581,#9105,.T.);
#24333=EDGE_CURVE('',#18582,#18583,#9106,.T.);
#24334=EDGE_CURVE('',#18582,#18458,#12463,.T.);
#24335=EDGE_CURVE('',#18457,#18456,#10273,.T.);
#24336=EDGE_CURVE('',#18583,#18455,#12464,.T.);
#24337=EDGE_CURVE('',#18584,#18585,#9107,.T.);
#24338=EDGE_CURVE('',#18585,#18586,#12465,.T.);
#24339=EDGE_CURVE('',#18586,#18587,#9108,.T.);
#24340=EDGE_CURVE('',#18587,#18584,#12466,.T.);
#24341=EDGE_CURVE('',#18585,#18584,#9109,.T.);
#24342=EDGE_CURVE('',#18586,#18587,#9110,.T.);
#24343=EDGE_CURVE('',#18588,#18589,#9111,.T.);
#24344=EDGE_CURVE('',#18588,#18462,#12467,.T.);
#24345=EDGE_CURVE('',#18461,#18460,#10274,.T.);
#24346=EDGE_CURVE('',#18589,#18459,#12468,.T.);
#24347=EDGE_CURVE('',#18590,#18591,#9112,.T.);
#24348=EDGE_CURVE('',#18591,#18592,#12469,.T.);
#24349=EDGE_CURVE('',#18592,#18593,#9113,.T.);
#24350=EDGE_CURVE('',#18593,#18590,#12470,.T.);
#24351=EDGE_CURVE('',#18591,#18590,#9114,.T.);
#24352=EDGE_CURVE('',#18592,#18593,#9115,.T.);
#24353=EDGE_CURVE('',#18594,#18595,#9116,.T.);
#24354=EDGE_CURVE('',#18594,#18466,#12471,.T.);
#24355=EDGE_CURVE('',#18465,#18464,#10275,.T.);
#24356=EDGE_CURVE('',#18595,#18463,#12472,.T.);
#24357=EDGE_CURVE('',#18596,#18597,#9117,.T.);
#24358=EDGE_CURVE('',#18597,#18598,#12473,.T.);
#24359=EDGE_CURVE('',#18598,#18599,#9118,.T.);
#24360=EDGE_CURVE('',#18599,#18596,#12474,.T.);
#24361=EDGE_CURVE('',#18597,#18596,#9119,.T.);
#24362=EDGE_CURVE('',#18598,#18599,#9120,.T.);
#24363=EDGE_CURVE('',#18600,#18601,#9121,.T.);
#24364=EDGE_CURVE('',#18600,#18470,#12475,.T.);
#24365=EDGE_CURVE('',#18469,#18468,#10276,.T.);
#24366=EDGE_CURVE('',#18601,#18467,#12476,.T.);
#24367=EDGE_CURVE('',#18602,#18603,#9122,.T.);
#24368=EDGE_CURVE('',#18603,#18604,#12477,.T.);
#24369=EDGE_CURVE('',#18604,#18605,#9123,.T.);
#24370=EDGE_CURVE('',#18605,#18602,#12478,.T.);
#24371=EDGE_CURVE('',#18603,#18602,#9124,.T.);
#24372=EDGE_CURVE('',#18604,#18605,#9125,.T.);
#24373=EDGE_CURVE('',#18606,#18607,#9126,.T.);
#24374=EDGE_CURVE('',#18606,#18474,#12479,.T.);
#24375=EDGE_CURVE('',#18473,#18472,#10277,.T.);
#24376=EDGE_CURVE('',#18607,#18471,#12480,.T.);
#24377=EDGE_CURVE('',#18608,#18609,#9127,.T.);
#24378=EDGE_CURVE('',#18609,#18610,#12481,.T.);
#24379=EDGE_CURVE('',#18610,#18611,#9128,.T.);
#24380=EDGE_CURVE('',#18611,#18608,#12482,.T.);
#24381=EDGE_CURVE('',#18609,#18608,#9129,.T.);
#24382=EDGE_CURVE('',#18610,#18611,#9130,.T.);
#24383=EDGE_CURVE('',#18612,#18613,#9131,.T.);
#24384=EDGE_CURVE('',#18612,#18478,#12483,.T.);
#24385=EDGE_CURVE('',#18477,#18476,#10278,.T.);
#24386=EDGE_CURVE('',#18613,#18475,#12484,.T.);
#24387=EDGE_CURVE('',#18614,#18615,#9132,.T.);
#24388=EDGE_CURVE('',#18615,#18616,#12485,.T.);
#24389=EDGE_CURVE('',#18616,#18617,#9133,.T.);
#24390=EDGE_CURVE('',#18617,#18614,#12486,.T.);
#24391=EDGE_CURVE('',#18615,#18614,#9134,.T.);
#24392=EDGE_CURVE('',#18616,#18617,#9135,.T.);
#24393=EDGE_CURVE('',#18618,#18619,#9136,.T.);
#24394=EDGE_CURVE('',#18618,#18482,#12487,.T.);
#24395=EDGE_CURVE('',#18481,#18480,#10279,.T.);
#24396=EDGE_CURVE('',#18619,#18479,#12488,.T.);
#24397=EDGE_CURVE('',#18620,#18621,#9137,.T.);
#24398=EDGE_CURVE('',#18621,#18622,#12489,.T.);
#24399=EDGE_CURVE('',#18622,#18623,#9138,.T.);
#24400=EDGE_CURVE('',#18623,#18620,#12490,.T.);
#24401=EDGE_CURVE('',#18621,#18620,#9139,.T.);
#24402=EDGE_CURVE('',#18622,#18623,#9140,.T.);
#24403=EDGE_CURVE('',#18624,#18625,#9141,.T.);
#24404=EDGE_CURVE('',#18624,#18486,#12491,.T.);
#24405=EDGE_CURVE('',#18485,#18484,#10280,.T.);
#24406=EDGE_CURVE('',#18625,#18483,#12492,.T.);
#24407=EDGE_CURVE('',#18626,#18627,#9142,.T.);
#24408=EDGE_CURVE('',#18627,#18628,#12493,.T.);
#24409=EDGE_CURVE('',#18628,#18629,#9143,.T.);
#24410=EDGE_CURVE('',#18629,#18626,#12494,.T.);
#24411=EDGE_CURVE('',#18627,#18626,#9144,.T.);
#24412=EDGE_CURVE('',#18628,#18629,#9145,.T.);
#24413=EDGE_CURVE('',#18630,#18631,#9146,.T.);
#24414=EDGE_CURVE('',#18630,#18490,#12495,.T.);
#24415=EDGE_CURVE('',#18489,#18488,#10281,.T.);
#24416=EDGE_CURVE('',#18631,#18487,#12496,.T.);
#24417=EDGE_CURVE('',#18632,#18633,#9147,.T.);
#24418=EDGE_CURVE('',#18633,#18634,#12497,.T.);
#24419=EDGE_CURVE('',#18634,#18635,#9148,.T.);
#24420=EDGE_CURVE('',#18635,#18632,#12498,.T.);
#24421=EDGE_CURVE('',#18633,#18632,#9149,.T.);
#24422=EDGE_CURVE('',#18634,#18635,#9150,.T.);
#24423=EDGE_CURVE('',#18636,#18637,#9151,.T.);
#24424=EDGE_CURVE('',#18636,#18494,#12499,.T.);
#24425=EDGE_CURVE('',#18493,#18492,#10282,.T.);
#24426=EDGE_CURVE('',#18637,#18491,#12500,.T.);
#24427=EDGE_CURVE('',#18638,#18639,#9152,.T.);
#24428=EDGE_CURVE('',#18639,#18640,#12501,.T.);
#24429=EDGE_CURVE('',#18640,#18641,#9153,.T.);
#24430=EDGE_CURVE('',#18641,#18638,#12502,.T.);
#24431=EDGE_CURVE('',#18639,#18638,#9154,.T.);
#24432=EDGE_CURVE('',#18640,#18641,#9155,.T.);
#24433=EDGE_CURVE('',#18642,#18643,#9156,.T.);
#24434=EDGE_CURVE('',#18642,#18498,#12503,.T.);
#24435=EDGE_CURVE('',#18497,#18496,#10283,.T.);
#24436=EDGE_CURVE('',#18643,#18495,#12504,.T.);
#24437=EDGE_CURVE('',#18644,#18645,#9157,.T.);
#24438=EDGE_CURVE('',#18645,#18646,#12505,.T.);
#24439=EDGE_CURVE('',#18646,#18647,#9158,.T.);
#24440=EDGE_CURVE('',#18647,#18644,#12506,.T.);
#24441=EDGE_CURVE('',#18645,#18644,#9159,.T.);
#24442=EDGE_CURVE('',#18646,#18647,#9160,.T.);
#24443=EDGE_CURVE('',#18648,#18649,#9161,.T.);
#24444=EDGE_CURVE('',#18648,#18506,#12507,.T.);
#24445=EDGE_CURVE('',#18505,#18504,#10284,.T.);
#24446=EDGE_CURVE('',#18649,#18503,#12508,.T.);
#24447=EDGE_CURVE('',#18650,#18651,#9162,.T.);
#24448=EDGE_CURVE('',#18651,#18652,#12509,.T.);
#24449=EDGE_CURVE('',#18652,#18653,#9163,.T.);
#24450=EDGE_CURVE('',#18653,#18650,#12510,.T.);
#24451=EDGE_CURVE('',#18651,#18650,#9164,.T.);
#24452=EDGE_CURVE('',#18652,#18653,#9165,.T.);
#24453=EDGE_CURVE('',#18654,#18655,#9166,.T.);
#24454=EDGE_CURVE('',#18654,#18502,#12511,.T.);
#24455=EDGE_CURVE('',#18501,#18500,#10285,.T.);
#24456=EDGE_CURVE('',#18655,#18499,#12512,.T.);
#24457=EDGE_CURVE('',#18656,#18657,#9167,.T.);
#24458=EDGE_CURVE('',#18657,#18658,#12513,.T.);
#24459=EDGE_CURVE('',#18658,#18659,#9168,.T.);
#24460=EDGE_CURVE('',#18659,#18656,#12514,.T.);
#24461=EDGE_CURVE('',#18657,#18656,#9169,.T.);
#24462=EDGE_CURVE('',#18658,#18659,#9170,.T.);
#24463=EDGE_CURVE('',#18404,#18660,#9171,.T.);
#24464=EDGE_CURVE('',#18660,#18661,#9172,.T.);
#24465=EDGE_CURVE('',#18661,#18662,#9173,.T.);
#24466=EDGE_CURVE('',#18662,#18661,#9174,.T.);
#24467=EDGE_CURVE('',#18660,#18508,#9175,.T.);
#24468=EDGE_CURVE('',#18406,#18509,#9176,.T.);
#24469=EDGE_CURVE('',#18405,#18507,#9177,.T.);
#24470=EDGE_CURVE('',#18396,#18648,#12515,.T.);
#24471=EDGE_CURVE('',#18649,#18654,#12516,.T.);
#24472=EDGE_CURVE('',#18655,#18642,#12517,.T.);
#24473=EDGE_CURVE('',#18643,#18636,#12518,.T.);
#24474=EDGE_CURVE('',#18637,#18630,#12519,.T.);
#24475=EDGE_CURVE('',#18631,#18624,#12520,.T.);
#24476=EDGE_CURVE('',#18625,#18618,#12521,.T.);
#24477=EDGE_CURVE('',#18619,#18612,#12522,.T.);
#24478=EDGE_CURVE('',#18613,#18606,#12523,.T.);
#24479=EDGE_CURVE('',#18607,#18600,#12524,.T.);
#24480=EDGE_CURVE('',#18601,#18594,#12525,.T.);
#24481=EDGE_CURVE('',#18595,#18588,#12526,.T.);
#24482=EDGE_CURVE('',#18589,#18582,#12527,.T.);
#24483=EDGE_CURVE('',#18583,#18576,#12528,.T.);
#24484=EDGE_CURVE('',#18577,#18570,#12529,.T.);
#24485=EDGE_CURVE('',#18571,#18564,#12530,.T.);
#24486=EDGE_CURVE('',#18565,#18558,#12531,.T.);
#24487=EDGE_CURVE('',#18559,#18552,#12532,.T.);
#24488=EDGE_CURVE('',#18553,#18546,#12533,.T.);
#24489=EDGE_CURVE('',#18547,#18540,#12534,.T.);
#24490=EDGE_CURVE('',#18541,#18534,#12535,.T.);
#24491=EDGE_CURVE('',#18535,#18528,#12536,.T.);
#24492=EDGE_CURVE('',#18529,#18522,#12537,.T.);
#24493=EDGE_CURVE('',#18523,#18516,#12538,.T.);
#24494=EDGE_CURVE('',#18517,#18510,#12539,.T.);
#24495=EDGE_CURVE('',#18511,#18397,#12540,.T.);
#24496=EDGE_CURVE('',#18662,#18306,#12541,.T.);
#24497=EDGE_CURVE('',#18335,#18340,#9178,.T.);
#24498=EDGE_CURVE('',#18314,#18373,#12542,.T.);
#34861=ORIENTED_EDGE('',*,*,#23942,.T.);
#34862=ORIENTED_EDGE('',*,*,#23943,.T.);
#34863=ORIENTED_EDGE('',*,*,#23944,.T.);
#34864=ORIENTED_EDGE('',*,*,#23945,.T.);
#34865=ORIENTED_EDGE('',*,*,#23943,.F.);
#34866=ORIENTED_EDGE('',*,*,#23945,.F.);
#34867=ORIENTED_EDGE('',*,*,#23946,.T.);
#34868=ORIENTED_EDGE('',*,*,#23947,.T.);
#34869=ORIENTED_EDGE('',*,*,#23946,.F.);
#34870=ORIENTED_EDGE('',*,*,#23944,.F.);
#34871=ORIENTED_EDGE('',*,*,#23942,.F.);
#34872=ORIENTED_EDGE('',*,*,#23948,.F.);
#34873=ORIENTED_EDGE('',*,*,#23949,.T.);
#34874=ORIENTED_EDGE('',*,*,#23950,.T.);
#34875=ORIENTED_EDGE('',*,*,#23951,.T.);
#34876=ORIENTED_EDGE('',*,*,#23952,.T.);
#34877=ORIENTED_EDGE('',*,*,#23950,.F.);
#34878=ORIENTED_EDGE('',*,*,#23952,.F.);
#34879=ORIENTED_EDGE('',*,*,#23953,.T.);
#34880=ORIENTED_EDGE('',*,*,#23954,.T.);
#34881=ORIENTED_EDGE('',*,*,#23953,.F.);
#34882=ORIENTED_EDGE('',*,*,#23951,.F.);
#34883=ORIENTED_EDGE('',*,*,#23949,.F.);
#34884=ORIENTED_EDGE('',*,*,#23947,.F.);
#34885=ORIENTED_EDGE('',*,*,#23955,.T.);
#34886=ORIENTED_EDGE('',*,*,#23956,.T.);
#34887=ORIENTED_EDGE('',*,*,#23957,.T.);
#34888=ORIENTED_EDGE('',*,*,#23958,.T.);
#34889=ORIENTED_EDGE('',*,*,#23956,.F.);
#34890=ORIENTED_EDGE('',*,*,#23958,.F.);
#34891=ORIENTED_EDGE('',*,*,#23959,.T.);
#34892=ORIENTED_EDGE('',*,*,#23960,.T.);
#34893=ORIENTED_EDGE('',*,*,#23959,.F.);
#34894=ORIENTED_EDGE('',*,*,#23957,.F.);
#34895=ORIENTED_EDGE('',*,*,#23955,.F.);
#34896=ORIENTED_EDGE('',*,*,#23954,.F.);
#34897=ORIENTED_EDGE('',*,*,#23961,.T.);
#34898=ORIENTED_EDGE('',*,*,#23962,.T.);
#34899=ORIENTED_EDGE('',*,*,#23963,.T.);
#34900=ORIENTED_EDGE('',*,*,#23964,.T.);
#34901=ORIENTED_EDGE('',*,*,#23965,.T.);
#34902=ORIENTED_EDGE('',*,*,#23963,.F.);
#34903=ORIENTED_EDGE('',*,*,#23965,.F.);
#34904=ORIENTED_EDGE('',*,*,#23966,.T.);
#34905=ORIENTED_EDGE('',*,*,#23967,.F.);
#34906=ORIENTED_EDGE('',*,*,#23968,.F.);
#34907=ORIENTED_EDGE('',*,*,#23966,.F.);
#34908=ORIENTED_EDGE('',*,*,#23964,.F.);
#34909=ORIENTED_EDGE('',*,*,#23969,.F.);
#34910=ORIENTED_EDGE('',*,*,#23970,.F.);
#34911=ORIENTED_EDGE('',*,*,#23971,.F.);
#34912=ORIENTED_EDGE('',*,*,#23972,.F.);
#34913=ORIENTED_EDGE('',*,*,#23973,.F.);
#34914=ORIENTED_EDGE('',*,*,#23974,.F.);
#34915=ORIENTED_EDGE('',*,*,#23975,.T.);
#34916=ORIENTED_EDGE('',*,*,#23961,.F.);
#34917=ORIENTED_EDGE('',*,*,#23962,.F.);
#34918=ORIENTED_EDGE('',*,*,#23975,.F.);
#34919=ORIENTED_EDGE('',*,*,#23976,.F.);
#34920=ORIENTED_EDGE('',*,*,#23967,.T.);
#34921=ORIENTED_EDGE('',*,*,#23968,.T.);
#34922=ORIENTED_EDGE('',*,*,#23977,.T.);
#34923=ORIENTED_EDGE('',*,*,#23978,.T.);
#34924=ORIENTED_EDGE('',*,*,#23979,.T.);
#34925=ORIENTED_EDGE('',*,*,#23977,.F.);
#34926=ORIENTED_EDGE('',*,*,#23979,.F.);
#34927=ORIENTED_EDGE('',*,*,#23980,.T.);
#34928=ORIENTED_EDGE('',*,*,#23981,.F.);
#34929=ORIENTED_EDGE('',*,*,#23982,.F.);
#34930=ORIENTED_EDGE('',*,*,#23980,.F.);
#34931=ORIENTED_EDGE('',*,*,#23978,.F.);
#34932=ORIENTED_EDGE('',*,*,#23983,.T.);
#34933=ORIENTED_EDGE('',*,*,#23984,.T.);
#34934=ORIENTED_EDGE('',*,*,#23985,.T.);
#34935=ORIENTED_EDGE('',*,*,#23986,.T.);
#34936=ORIENTED_EDGE('',*,*,#23987,.T.);
#34937=ORIENTED_EDGE('',*,*,#23988,.T.);
#34938=ORIENTED_EDGE('',*,*,#23989,.T.);
#34939=ORIENTED_EDGE('',*,*,#23990,.T.);
#34940=ORIENTED_EDGE('',*,*,#23987,.F.);
#34941=ORIENTED_EDGE('',*,*,#23991,.T.);
#34942=ORIENTED_EDGE('',*,*,#23983,.F.);
#34943=ORIENTED_EDGE('',*,*,#23992,.T.);
#34944=ORIENTED_EDGE('',*,*,#23993,.T.);
#34945=ORIENTED_EDGE('',*,*,#23994,.T.);
#34946=ORIENTED_EDGE('',*,*,#23995,.T.);
#34947=ORIENTED_EDGE('',*,*,#23992,.F.);
#34948=ORIENTED_EDGE('',*,*,#23996,.T.);
#34949=ORIENTED_EDGE('',*,*,#23989,.F.);
#34950=ORIENTED_EDGE('',*,*,#23984,.F.);
#34951=ORIENTED_EDGE('',*,*,#23997,.F.);
#34952=ORIENTED_EDGE('',*,*,#23998,.F.);
#34953=ORIENTED_EDGE('',*,*,#23999,.T.);
#34954=ORIENTED_EDGE('',*,*,#23991,.F.);
#34955=ORIENTED_EDGE('',*,*,#24000,.T.);
#34956=ORIENTED_EDGE('',*,*,#24001,.T.);
#34957=ORIENTED_EDGE('',*,*,#23997,.T.);
#34958=ORIENTED_EDGE('',*,*,#24002,.F.);
#34959=ORIENTED_EDGE('',*,*,#23990,.F.);
#34960=ORIENTED_EDGE('',*,*,#24003,.F.);
#34961=ORIENTED_EDGE('',*,*,#24004,.F.);
#34962=ORIENTED_EDGE('',*,*,#24005,.F.);
#34963=ORIENTED_EDGE('',*,*,#24006,.F.);
#34964=ORIENTED_EDGE('',*,*,#24000,.F.);
#34965=ORIENTED_EDGE('',*,*,#23996,.F.);
#34966=ORIENTED_EDGE('',*,*,#24007,.T.);
#34967=ORIENTED_EDGE('',*,*,#24008,.T.);
#34968=ORIENTED_EDGE('',*,*,#24003,.T.);
#34969=ORIENTED_EDGE('',*,*,#23995,.F.);
#34970=ORIENTED_EDGE('',*,*,#24009,.T.);
#34971=ORIENTED_EDGE('',*,*,#24010,.F.);
#34972=ORIENTED_EDGE('',*,*,#24007,.F.);
#34973=ORIENTED_EDGE('',*,*,#24011,.T.);
#34974=ORIENTED_EDGE('',*,*,#24012,.T.);
#34975=ORIENTED_EDGE('',*,*,#24013,.T.);
#34976=ORIENTED_EDGE('',*,*,#23998,.T.);
#34977=ORIENTED_EDGE('',*,*,#24001,.F.);
#34978=ORIENTED_EDGE('',*,*,#24014,.T.);
#34979=ORIENTED_EDGE('',*,*,#24011,.F.);
#34980=ORIENTED_EDGE('',*,*,#24012,.F.);
#34981=ORIENTED_EDGE('',*,*,#24015,.F.);
#34982=ORIENTED_EDGE('',*,*,#24016,.F.);
#34983=ORIENTED_EDGE('',*,*,#24017,.T.);
#34984=ORIENTED_EDGE('',*,*,#24014,.F.);
#34985=ORIENTED_EDGE('',*,*,#24006,.T.);
#34986=ORIENTED_EDGE('',*,*,#24018,.T.);
#34987=ORIENTED_EDGE('',*,*,#24015,.T.);
#34988=ORIENTED_EDGE('',*,*,#23981,.T.);
#34989=ORIENTED_EDGE('',*,*,#23982,.T.);
#34990=ORIENTED_EDGE('',*,*,#24019,.T.);
#34991=ORIENTED_EDGE('',*,*,#24002,.T.);
#34992=ORIENTED_EDGE('',*,*,#24019,.F.);
#34993=ORIENTED_EDGE('',*,*,#24020,.F.);
#34994=ORIENTED_EDGE('',*,*,#24021,.T.);
#34995=ORIENTED_EDGE('',*,*,#24022,.T.);
#34996=ORIENTED_EDGE('',*,*,#24023,.T.);
#34997=ORIENTED_EDGE('',*,*,#24023,.F.);
#34998=ORIENTED_EDGE('',*,*,#24024,.F.);
#34999=ORIENTED_EDGE('',*,*,#24025,.T.);
#35000=ORIENTED_EDGE('',*,*,#24026,.F.);
#35001=ORIENTED_EDGE('',*,*,#24027,.F.);
#35002=ORIENTED_EDGE('',*,*,#24028,.F.);
#35003=ORIENTED_EDGE('',*,*,#24029,.F.);
#35004=ORIENTED_EDGE('',*,*,#24030,.F.);
#35005=ORIENTED_EDGE('',*,*,#24031,.F.);
#35006=ORIENTED_EDGE('',*,*,#24032,.T.);
#35007=ORIENTED_EDGE('',*,*,#24033,.T.);
#35008=ORIENTED_EDGE('',*,*,#24027,.T.);
#35009=ORIENTED_EDGE('',*,*,#24034,.T.);
#35010=ORIENTED_EDGE('',*,*,#24010,.T.);
#35011=ORIENTED_EDGE('',*,*,#24035,.T.);
#35012=ORIENTED_EDGE('',*,*,#24036,.T.);
#35013=ORIENTED_EDGE('',*,*,#24034,.F.);
#35014=ORIENTED_EDGE('',*,*,#24037,.T.);
#35015=ORIENTED_EDGE('',*,*,#24008,.F.);
#35016=ORIENTED_EDGE('',*,*,#24037,.F.);
#35017=ORIENTED_EDGE('',*,*,#24038,.T.);
#35018=ORIENTED_EDGE('',*,*,#24039,.T.);
#35019=ORIENTED_EDGE('',*,*,#24004,.T.);
#35020=ORIENTED_EDGE('',*,*,#24036,.F.);
#35021=ORIENTED_EDGE('',*,*,#24040,.T.);
#35022=ORIENTED_EDGE('',*,*,#24041,.F.);
#35023=ORIENTED_EDGE('',*,*,#24038,.F.);
#35024=ORIENTED_EDGE('',*,*,#24042,.T.);
#35025=ORIENTED_EDGE('',*,*,#24043,.T.);
#35026=ORIENTED_EDGE('',*,*,#24044,.T.);
#35027=ORIENTED_EDGE('',*,*,#24016,.T.);
#35028=ORIENTED_EDGE('',*,*,#24018,.F.);
#35029=ORIENTED_EDGE('',*,*,#24045,.T.);
#35030=ORIENTED_EDGE('',*,*,#24042,.F.);
#35031=ORIENTED_EDGE('',*,*,#24045,.F.);
#35032=ORIENTED_EDGE('',*,*,#24005,.T.);
#35033=ORIENTED_EDGE('',*,*,#24046,.T.);
#35034=ORIENTED_EDGE('',*,*,#24047,.T.);
#35035=ORIENTED_EDGE('',*,*,#24039,.F.);
#35036=ORIENTED_EDGE('',*,*,#24048,.T.);
#35037=ORIENTED_EDGE('',*,*,#24046,.F.);
#35038=ORIENTED_EDGE('',*,*,#24043,.F.);
#35039=ORIENTED_EDGE('',*,*,#24047,.F.);
#35040=ORIENTED_EDGE('',*,*,#24049,.F.);
#35041=ORIENTED_EDGE('',*,*,#24050,.T.);
#35042=ORIENTED_EDGE('',*,*,#24048,.F.);
#35043=ORIENTED_EDGE('',*,*,#24041,.T.);
#35044=ORIENTED_EDGE('',*,*,#24051,.T.);
#35045=ORIENTED_EDGE('',*,*,#24049,.T.);
#35046=ORIENTED_EDGE('',*,*,#24026,.T.);
#35047=ORIENTED_EDGE('',*,*,#24052,.T.);
#35048=ORIENTED_EDGE('',*,*,#24024,.T.);
#35049=ORIENTED_EDGE('',*,*,#24022,.F.);
#35050=ORIENTED_EDGE('',*,*,#24053,.F.);
#35051=ORIENTED_EDGE('',*,*,#24054,.F.);
#35052=ORIENTED_EDGE('',*,*,#24031,.T.);
#35053=ORIENTED_EDGE('',*,*,#24052,.F.);
#35054=ORIENTED_EDGE('',*,*,#24025,.F.);
#35055=ORIENTED_EDGE('',*,*,#24032,.F.);
#35056=ORIENTED_EDGE('',*,*,#24055,.F.);
#35057=ORIENTED_EDGE('',*,*,#24056,.F.);
#35058=ORIENTED_EDGE('',*,*,#23969,.T.);
#35059=ORIENTED_EDGE('',*,*,#24030,.T.);
#35060=ORIENTED_EDGE('',*,*,#24057,.T.);
#35061=ORIENTED_EDGE('',*,*,#24028,.T.);
#35062=ORIENTED_EDGE('',*,*,#24033,.F.);
#35063=ORIENTED_EDGE('',*,*,#23976,.T.);
#35064=ORIENTED_EDGE('',*,*,#23974,.T.);
#35065=ORIENTED_EDGE('',*,*,#24020,.T.);
#35066=ORIENTED_EDGE('',*,*,#24057,.F.);
#35067=ORIENTED_EDGE('',*,*,#24029,.T.);
#35068=ORIENTED_EDGE('',*,*,#23972,.T.);
#35069=ORIENTED_EDGE('',*,*,#24058,.T.);
#35070=ORIENTED_EDGE('',*,*,#24059,.T.);
#35071=ORIENTED_EDGE('',*,*,#24060,.T.);
#35072=ORIENTED_EDGE('',*,*,#24061,.T.);
#35073=ORIENTED_EDGE('',*,*,#24062,.T.);
#35074=ORIENTED_EDGE('',*,*,#24063,.T.);
#35075=ORIENTED_EDGE('',*,*,#24058,.F.);
#35076=ORIENTED_EDGE('',*,*,#24064,.T.);
#35077=ORIENTED_EDGE('',*,*,#24065,.T.);
#35078=ORIENTED_EDGE('',*,*,#24066,.T.);
#35079=ORIENTED_EDGE('',*,*,#24067,.T.);
#35080=ORIENTED_EDGE('',*,*,#24068,.T.);
#35081=ORIENTED_EDGE('',*,*,#24062,.F.);
#35082=ORIENTED_EDGE('',*,*,#24069,.F.);
#35083=ORIENTED_EDGE('',*,*,#24067,.F.);
#35084=ORIENTED_EDGE('',*,*,#24070,.T.);
#35085=ORIENTED_EDGE('',*,*,#24071,.T.);
#35086=ORIENTED_EDGE('',*,*,#24072,.T.);
#35087=ORIENTED_EDGE('',*,*,#24065,.F.);
#35088=ORIENTED_EDGE('',*,*,#24066,.F.);
#35089=ORIENTED_EDGE('',*,*,#24061,.F.);
#35090=ORIENTED_EDGE('',*,*,#24073,.F.);
#35091=ORIENTED_EDGE('',*,*,#24059,.F.);
#35092=ORIENTED_EDGE('',*,*,#24063,.F.);
#35093=ORIENTED_EDGE('',*,*,#24072,.F.);
#35094=ORIENTED_EDGE('',*,*,#24074,.T.);
#35095=ORIENTED_EDGE('',*,*,#24070,.F.);
#35096=ORIENTED_EDGE('',*,*,#24060,.F.);
#35097=ORIENTED_EDGE('',*,*,#24073,.T.);
#35098=ORIENTED_EDGE('',*,*,#24021,.F.);
#35099=ORIENTED_EDGE('',*,*,#23973,.T.);
#35100=ORIENTED_EDGE('',*,*,#24068,.F.);
#35101=ORIENTED_EDGE('',*,*,#24075,.F.);
#35102=ORIENTED_EDGE('',*,*,#24064,.F.);
#35103=ORIENTED_EDGE('',*,*,#23971,.T.);
#35104=ORIENTED_EDGE('',*,*,#24076,.F.);
#35105=ORIENTED_EDGE('',*,*,#24077,.F.);
#35106=ORIENTED_EDGE('',*,*,#23970,.T.);
#35107=ORIENTED_EDGE('',*,*,#24078,.T.);
#35108=ORIENTED_EDGE('',*,*,#24079,.T.);
#35109=ORIENTED_EDGE('',*,*,#24080,.T.);
#35110=ORIENTED_EDGE('',*,*,#24081,.T.);
#35111=ORIENTED_EDGE('',*,*,#24082,.T.);
#35112=ORIENTED_EDGE('',*,*,#24083,.T.);
#35113=ORIENTED_EDGE('',*,*,#24078,.F.);
#35114=ORIENTED_EDGE('',*,*,#24056,.T.);
#35115=ORIENTED_EDGE('',*,*,#24084,.T.);
#35116=ORIENTED_EDGE('',*,*,#24085,.T.);
#35117=ORIENTED_EDGE('',*,*,#24086,.T.);
#35118=ORIENTED_EDGE('',*,*,#24076,.T.);
#35119=ORIENTED_EDGE('',*,*,#24082,.F.);
#35120=ORIENTED_EDGE('',*,*,#24087,.F.);
#35121=ORIENTED_EDGE('',*,*,#24086,.F.);
#35122=ORIENTED_EDGE('',*,*,#24088,.T.);
#35123=ORIENTED_EDGE('',*,*,#24089,.T.);
#35124=ORIENTED_EDGE('',*,*,#24090,.T.);
#35125=ORIENTED_EDGE('',*,*,#24084,.F.);
#35126=ORIENTED_EDGE('',*,*,#24085,.F.);
#35127=ORIENTED_EDGE('',*,*,#24081,.F.);
#35128=ORIENTED_EDGE('',*,*,#24091,.F.);
#35129=ORIENTED_EDGE('',*,*,#24079,.F.);
#35130=ORIENTED_EDGE('',*,*,#24083,.F.);
#35131=ORIENTED_EDGE('',*,*,#24090,.F.);
#35132=ORIENTED_EDGE('',*,*,#24092,.T.);
#35133=ORIENTED_EDGE('',*,*,#24088,.F.);
#35134=ORIENTED_EDGE('',*,*,#24080,.F.);
#35135=ORIENTED_EDGE('',*,*,#24091,.T.);
#35136=ORIENTED_EDGE('',*,*,#24093,.T.);
#35137=ORIENTED_EDGE('',*,*,#24094,.F.);
#35138=ORIENTED_EDGE('',*,*,#24095,.T.);
#35139=ORIENTED_EDGE('',*,*,#24096,.T.);
#35140=ORIENTED_EDGE('',*,*,#24097,.T.);
#35141=ORIENTED_EDGE('',*,*,#24098,.T.);
#35142=ORIENTED_EDGE('',*,*,#24099,.T.);
#35143=ORIENTED_EDGE('',*,*,#24100,.T.);
#35144=ORIENTED_EDGE('',*,*,#24101,.T.);
#35145=ORIENTED_EDGE('',*,*,#24102,.T.);
#35146=ORIENTED_EDGE('',*,*,#24100,.F.);
#35147=ORIENTED_EDGE('',*,*,#24103,.T.);
#35148=ORIENTED_EDGE('',*,*,#24102,.F.);
#35149=ORIENTED_EDGE('',*,*,#24104,.F.);
#35150=ORIENTED_EDGE('',*,*,#24099,.F.);
#35151=ORIENTED_EDGE('',*,*,#24103,.F.);
#35152=ORIENTED_EDGE('',*,*,#24105,.F.);
#35153=ORIENTED_EDGE('',*,*,#24106,.T.);
#35154=ORIENTED_EDGE('',*,*,#24107,.T.);
#35155=ORIENTED_EDGE('',*,*,#24093,.F.);
#35156=ORIENTED_EDGE('',*,*,#24108,.T.);
#35157=ORIENTED_EDGE('',*,*,#24097,.F.);
#35158=ORIENTED_EDGE('',*,*,#24109,.T.);
#35159=ORIENTED_EDGE('',*,*,#24110,.F.);
#35160=ORIENTED_EDGE('',*,*,#24111,.T.);
#35161=ORIENTED_EDGE('',*,*,#24112,.F.);
#35162=ORIENTED_EDGE('',*,*,#24113,.T.);
#35163=ORIENTED_EDGE('',*,*,#24114,.F.);
#35164=ORIENTED_EDGE('',*,*,#24115,.T.);
#35165=ORIENTED_EDGE('',*,*,#24116,.F.);
#35166=ORIENTED_EDGE('',*,*,#24117,.T.);
#35167=ORIENTED_EDGE('',*,*,#24118,.F.);
#35168=ORIENTED_EDGE('',*,*,#24119,.T.);
#35169=ORIENTED_EDGE('',*,*,#24120,.F.);
#35170=ORIENTED_EDGE('',*,*,#24121,.T.);
#35171=ORIENTED_EDGE('',*,*,#24122,.F.);
#35172=ORIENTED_EDGE('',*,*,#24123,.T.);
#35173=ORIENTED_EDGE('',*,*,#24124,.F.);
#35174=ORIENTED_EDGE('',*,*,#24125,.T.);
#35175=ORIENTED_EDGE('',*,*,#24126,.F.);
#35176=ORIENTED_EDGE('',*,*,#24127,.T.);
#35177=ORIENTED_EDGE('',*,*,#24128,.F.);
#35178=ORIENTED_EDGE('',*,*,#24129,.T.);
#35179=ORIENTED_EDGE('',*,*,#24130,.F.);
#35180=ORIENTED_EDGE('',*,*,#24131,.T.);
#35181=ORIENTED_EDGE('',*,*,#24132,.F.);
#35182=ORIENTED_EDGE('',*,*,#24133,.T.);
#35183=ORIENTED_EDGE('',*,*,#24134,.F.);
#35184=ORIENTED_EDGE('',*,*,#24135,.T.);
#35185=ORIENTED_EDGE('',*,*,#24136,.F.);
#35186=ORIENTED_EDGE('',*,*,#24137,.T.);
#35187=ORIENTED_EDGE('',*,*,#24138,.F.);
#35188=ORIENTED_EDGE('',*,*,#24139,.T.);
#35189=ORIENTED_EDGE('',*,*,#24140,.F.);
#35190=ORIENTED_EDGE('',*,*,#24141,.T.);
#35191=ORIENTED_EDGE('',*,*,#24142,.F.);
#35192=ORIENTED_EDGE('',*,*,#24143,.T.);
#35193=ORIENTED_EDGE('',*,*,#24144,.F.);
#35194=ORIENTED_EDGE('',*,*,#24145,.T.);
#35195=ORIENTED_EDGE('',*,*,#24146,.F.);
#35196=ORIENTED_EDGE('',*,*,#24147,.T.);
#35197=ORIENTED_EDGE('',*,*,#24148,.F.);
#35198=ORIENTED_EDGE('',*,*,#24149,.T.);
#35199=ORIENTED_EDGE('',*,*,#24150,.F.);
#35200=ORIENTED_EDGE('',*,*,#24151,.T.);
#35201=ORIENTED_EDGE('',*,*,#24152,.F.);
#35202=ORIENTED_EDGE('',*,*,#24153,.T.);
#35203=ORIENTED_EDGE('',*,*,#24154,.F.);
#35204=ORIENTED_EDGE('',*,*,#24155,.T.);
#35205=ORIENTED_EDGE('',*,*,#24156,.F.);
#35206=ORIENTED_EDGE('',*,*,#24157,.T.);
#35207=ORIENTED_EDGE('',*,*,#24158,.F.);
#35208=ORIENTED_EDGE('',*,*,#24159,.T.);
#35209=ORIENTED_EDGE('',*,*,#24160,.F.);
#35210=ORIENTED_EDGE('',*,*,#24161,.T.);
#35211=ORIENTED_EDGE('',*,*,#24162,.F.);
#35212=ORIENTED_EDGE('',*,*,#24163,.T.);
#35213=ORIENTED_EDGE('',*,*,#24164,.F.);
#35214=ORIENTED_EDGE('',*,*,#24165,.T.);
#35215=ORIENTED_EDGE('',*,*,#24166,.F.);
#35216=ORIENTED_EDGE('',*,*,#24167,.T.);
#35217=ORIENTED_EDGE('',*,*,#24168,.F.);
#35218=ORIENTED_EDGE('',*,*,#24169,.T.);
#35219=ORIENTED_EDGE('',*,*,#24170,.F.);
#35220=ORIENTED_EDGE('',*,*,#24171,.T.);
#35221=ORIENTED_EDGE('',*,*,#24172,.F.);
#35222=ORIENTED_EDGE('',*,*,#24173,.T.);
#35223=ORIENTED_EDGE('',*,*,#24174,.F.);
#35224=ORIENTED_EDGE('',*,*,#24175,.T.);
#35225=ORIENTED_EDGE('',*,*,#24176,.F.);
#35226=ORIENTED_EDGE('',*,*,#24177,.T.);
#35227=ORIENTED_EDGE('',*,*,#24178,.F.);
#35228=ORIENTED_EDGE('',*,*,#24179,.T.);
#35229=ORIENTED_EDGE('',*,*,#24180,.F.);
#35230=ORIENTED_EDGE('',*,*,#24181,.T.);
#35231=ORIENTED_EDGE('',*,*,#24182,.F.);
#35232=ORIENTED_EDGE('',*,*,#24183,.T.);
#35233=ORIENTED_EDGE('',*,*,#24184,.F.);
#35234=ORIENTED_EDGE('',*,*,#24185,.T.);
#35235=ORIENTED_EDGE('',*,*,#24186,.F.);
#35236=ORIENTED_EDGE('',*,*,#24187,.T.);
#35237=ORIENTED_EDGE('',*,*,#24188,.F.);
#35238=ORIENTED_EDGE('',*,*,#24189,.T.);
#35239=ORIENTED_EDGE('',*,*,#24190,.F.);
#35240=ORIENTED_EDGE('',*,*,#24191,.T.);
#35241=ORIENTED_EDGE('',*,*,#24192,.F.);
#35242=ORIENTED_EDGE('',*,*,#24193,.T.);
#35243=ORIENTED_EDGE('',*,*,#24194,.F.);
#35244=ORIENTED_EDGE('',*,*,#24195,.T.);
#35245=ORIENTED_EDGE('',*,*,#24196,.F.);
#35246=ORIENTED_EDGE('',*,*,#24197,.T.);
#35247=ORIENTED_EDGE('',*,*,#24198,.F.);
#35248=ORIENTED_EDGE('',*,*,#24199,.T.);
#35249=ORIENTED_EDGE('',*,*,#24200,.F.);
#35250=ORIENTED_EDGE('',*,*,#24201,.T.);
#35251=ORIENTED_EDGE('',*,*,#24202,.F.);
#35252=ORIENTED_EDGE('',*,*,#24203,.T.);
#35253=ORIENTED_EDGE('',*,*,#24204,.F.);
#35254=ORIENTED_EDGE('',*,*,#24205,.T.);
#35255=ORIENTED_EDGE('',*,*,#24206,.F.);
#35256=ORIENTED_EDGE('',*,*,#24207,.T.);
#35257=ORIENTED_EDGE('',*,*,#24208,.F.);
#35258=ORIENTED_EDGE('',*,*,#24209,.T.);
#35259=ORIENTED_EDGE('',*,*,#24098,.F.);
#35260=ORIENTED_EDGE('',*,*,#24108,.F.);
#35261=ORIENTED_EDGE('',*,*,#24210,.F.);
#35262=ORIENTED_EDGE('',*,*,#24211,.T.);
#35263=ORIENTED_EDGE('',*,*,#24212,.T.);
#35264=ORIENTED_EDGE('',*,*,#24101,.F.);
#35265=ORIENTED_EDGE('',*,*,#24104,.T.);
#35266=ORIENTED_EDGE('',*,*,#24213,.F.);
#35267=ORIENTED_EDGE('',*,*,#24214,.T.);
#35268=ORIENTED_EDGE('',*,*,#24112,.T.);
#35269=ORIENTED_EDGE('',*,*,#24215,.T.);
#35270=ORIENTED_EDGE('',*,*,#24110,.T.);
#35271=ORIENTED_EDGE('',*,*,#24216,.F.);
#35272=ORIENTED_EDGE('',*,*,#24217,.T.);
#35273=ORIENTED_EDGE('',*,*,#24218,.T.);
#35274=ORIENTED_EDGE('',*,*,#24219,.T.);
#35275=ORIENTED_EDGE('',*,*,#24220,.T.);
#35276=ORIENTED_EDGE('',*,*,#24218,.F.);
#35277=ORIENTED_EDGE('',*,*,#24221,.T.);
#35278=ORIENTED_EDGE('',*,*,#24220,.F.);
#35279=ORIENTED_EDGE('',*,*,#24222,.F.);
#35280=ORIENTED_EDGE('',*,*,#24217,.F.);
#35281=ORIENTED_EDGE('',*,*,#24221,.F.);
#35282=ORIENTED_EDGE('',*,*,#24215,.F.);
#35283=ORIENTED_EDGE('',*,*,#24111,.F.);
#35284=ORIENTED_EDGE('',*,*,#24219,.F.);
#35285=ORIENTED_EDGE('',*,*,#24222,.T.);
#35286=ORIENTED_EDGE('',*,*,#24223,.F.);
#35287=ORIENTED_EDGE('',*,*,#24224,.T.);
#35288=ORIENTED_EDGE('',*,*,#24116,.T.);
#35289=ORIENTED_EDGE('',*,*,#24225,.T.);
#35290=ORIENTED_EDGE('',*,*,#24114,.T.);
#35291=ORIENTED_EDGE('',*,*,#24226,.F.);
#35292=ORIENTED_EDGE('',*,*,#24227,.T.);
#35293=ORIENTED_EDGE('',*,*,#24228,.T.);
#35294=ORIENTED_EDGE('',*,*,#24229,.T.);
#35295=ORIENTED_EDGE('',*,*,#24230,.T.);
#35296=ORIENTED_EDGE('',*,*,#24228,.F.);
#35297=ORIENTED_EDGE('',*,*,#24231,.T.);
#35298=ORIENTED_EDGE('',*,*,#24230,.F.);
#35299=ORIENTED_EDGE('',*,*,#24232,.F.);
#35300=ORIENTED_EDGE('',*,*,#24227,.F.);
#35301=ORIENTED_EDGE('',*,*,#24231,.F.);
#35302=ORIENTED_EDGE('',*,*,#24225,.F.);
#35303=ORIENTED_EDGE('',*,*,#24115,.F.);
#35304=ORIENTED_EDGE('',*,*,#24229,.F.);
#35305=ORIENTED_EDGE('',*,*,#24232,.T.);
#35306=ORIENTED_EDGE('',*,*,#24233,.F.);
#35307=ORIENTED_EDGE('',*,*,#24234,.T.);
#35308=ORIENTED_EDGE('',*,*,#24120,.T.);
#35309=ORIENTED_EDGE('',*,*,#24235,.T.);
#35310=ORIENTED_EDGE('',*,*,#24118,.T.);
#35311=ORIENTED_EDGE('',*,*,#24236,.F.);
#35312=ORIENTED_EDGE('',*,*,#24237,.T.);
#35313=ORIENTED_EDGE('',*,*,#24238,.T.);
#35314=ORIENTED_EDGE('',*,*,#24239,.T.);
#35315=ORIENTED_EDGE('',*,*,#24240,.T.);
#35316=ORIENTED_EDGE('',*,*,#24238,.F.);
#35317=ORIENTED_EDGE('',*,*,#24241,.T.);
#35318=ORIENTED_EDGE('',*,*,#24240,.F.);
#35319=ORIENTED_EDGE('',*,*,#24242,.F.);
#35320=ORIENTED_EDGE('',*,*,#24237,.F.);
#35321=ORIENTED_EDGE('',*,*,#24241,.F.);
#35322=ORIENTED_EDGE('',*,*,#24235,.F.);
#35323=ORIENTED_EDGE('',*,*,#24119,.F.);
#35324=ORIENTED_EDGE('',*,*,#24239,.F.);
#35325=ORIENTED_EDGE('',*,*,#24242,.T.);
#35326=ORIENTED_EDGE('',*,*,#24243,.F.);
#35327=ORIENTED_EDGE('',*,*,#24244,.T.);
#35328=ORIENTED_EDGE('',*,*,#24124,.T.);
#35329=ORIENTED_EDGE('',*,*,#24245,.T.);
#35330=ORIENTED_EDGE('',*,*,#24122,.T.);
#35331=ORIENTED_EDGE('',*,*,#24246,.F.);
#35332=ORIENTED_EDGE('',*,*,#24247,.T.);
#35333=ORIENTED_EDGE('',*,*,#24248,.T.);
#35334=ORIENTED_EDGE('',*,*,#24249,.T.);
#35335=ORIENTED_EDGE('',*,*,#24250,.T.);
#35336=ORIENTED_EDGE('',*,*,#24248,.F.);
#35337=ORIENTED_EDGE('',*,*,#24251,.T.);
#35338=ORIENTED_EDGE('',*,*,#24250,.F.);
#35339=ORIENTED_EDGE('',*,*,#24252,.F.);
#35340=ORIENTED_EDGE('',*,*,#24247,.F.);
#35341=ORIENTED_EDGE('',*,*,#24251,.F.);
#35342=ORIENTED_EDGE('',*,*,#24245,.F.);
#35343=ORIENTED_EDGE('',*,*,#24123,.F.);
#35344=ORIENTED_EDGE('',*,*,#24249,.F.);
#35345=ORIENTED_EDGE('',*,*,#24252,.T.);
#35346=ORIENTED_EDGE('',*,*,#24253,.F.);
#35347=ORIENTED_EDGE('',*,*,#24254,.T.);
#35348=ORIENTED_EDGE('',*,*,#24128,.T.);
#35349=ORIENTED_EDGE('',*,*,#24255,.T.);
#35350=ORIENTED_EDGE('',*,*,#24126,.T.);
#35351=ORIENTED_EDGE('',*,*,#24256,.F.);
#35352=ORIENTED_EDGE('',*,*,#24257,.T.);
#35353=ORIENTED_EDGE('',*,*,#24258,.T.);
#35354=ORIENTED_EDGE('',*,*,#24259,.T.);
#35355=ORIENTED_EDGE('',*,*,#24260,.T.);
#35356=ORIENTED_EDGE('',*,*,#24258,.F.);
#35357=ORIENTED_EDGE('',*,*,#24261,.T.);
#35358=ORIENTED_EDGE('',*,*,#24260,.F.);
#35359=ORIENTED_EDGE('',*,*,#24262,.F.);
#35360=ORIENTED_EDGE('',*,*,#24257,.F.);
#35361=ORIENTED_EDGE('',*,*,#24261,.F.);
#35362=ORIENTED_EDGE('',*,*,#24255,.F.);
#35363=ORIENTED_EDGE('',*,*,#24127,.F.);
#35364=ORIENTED_EDGE('',*,*,#24259,.F.);
#35365=ORIENTED_EDGE('',*,*,#24262,.T.);
#35366=ORIENTED_EDGE('',*,*,#24263,.F.);
#35367=ORIENTED_EDGE('',*,*,#24264,.T.);
#35368=ORIENTED_EDGE('',*,*,#24132,.T.);
#35369=ORIENTED_EDGE('',*,*,#24265,.T.);
#35370=ORIENTED_EDGE('',*,*,#24130,.T.);
#35371=ORIENTED_EDGE('',*,*,#24266,.F.);
#35372=ORIENTED_EDGE('',*,*,#24267,.T.);
#35373=ORIENTED_EDGE('',*,*,#24268,.T.);
#35374=ORIENTED_EDGE('',*,*,#24269,.T.);
#35375=ORIENTED_EDGE('',*,*,#24270,.T.);
#35376=ORIENTED_EDGE('',*,*,#24268,.F.);
#35377=ORIENTED_EDGE('',*,*,#24271,.T.);
#35378=ORIENTED_EDGE('',*,*,#24270,.F.);
#35379=ORIENTED_EDGE('',*,*,#24272,.F.);
#35380=ORIENTED_EDGE('',*,*,#24267,.F.);
#35381=ORIENTED_EDGE('',*,*,#24271,.F.);
#35382=ORIENTED_EDGE('',*,*,#24265,.F.);
#35383=ORIENTED_EDGE('',*,*,#24131,.F.);
#35384=ORIENTED_EDGE('',*,*,#24269,.F.);
#35385=ORIENTED_EDGE('',*,*,#24272,.T.);
#35386=ORIENTED_EDGE('',*,*,#24273,.F.);
#35387=ORIENTED_EDGE('',*,*,#24274,.T.);
#35388=ORIENTED_EDGE('',*,*,#24136,.T.);
#35389=ORIENTED_EDGE('',*,*,#24275,.T.);
#35390=ORIENTED_EDGE('',*,*,#24134,.T.);
#35391=ORIENTED_EDGE('',*,*,#24276,.F.);
#35392=ORIENTED_EDGE('',*,*,#24277,.T.);
#35393=ORIENTED_EDGE('',*,*,#24278,.T.);
#35394=ORIENTED_EDGE('',*,*,#24279,.T.);
#35395=ORIENTED_EDGE('',*,*,#24280,.T.);
#35396=ORIENTED_EDGE('',*,*,#24278,.F.);
#35397=ORIENTED_EDGE('',*,*,#24281,.T.);
#35398=ORIENTED_EDGE('',*,*,#24280,.F.);
#35399=ORIENTED_EDGE('',*,*,#24282,.F.);
#35400=ORIENTED_EDGE('',*,*,#24277,.F.);
#35401=ORIENTED_EDGE('',*,*,#24281,.F.);
#35402=ORIENTED_EDGE('',*,*,#24275,.F.);
#35403=ORIENTED_EDGE('',*,*,#24135,.F.);
#35404=ORIENTED_EDGE('',*,*,#24279,.F.);
#35405=ORIENTED_EDGE('',*,*,#24282,.T.);
#35406=ORIENTED_EDGE('',*,*,#24283,.F.);
#35407=ORIENTED_EDGE('',*,*,#24284,.T.);
#35408=ORIENTED_EDGE('',*,*,#24140,.T.);
#35409=ORIENTED_EDGE('',*,*,#24285,.T.);
#35410=ORIENTED_EDGE('',*,*,#24138,.T.);
#35411=ORIENTED_EDGE('',*,*,#24286,.F.);
#35412=ORIENTED_EDGE('',*,*,#24287,.T.);
#35413=ORIENTED_EDGE('',*,*,#24288,.T.);
#35414=ORIENTED_EDGE('',*,*,#24289,.T.);
#35415=ORIENTED_EDGE('',*,*,#24290,.T.);
#35416=ORIENTED_EDGE('',*,*,#24288,.F.);
#35417=ORIENTED_EDGE('',*,*,#24291,.T.);
#35418=ORIENTED_EDGE('',*,*,#24290,.F.);
#35419=ORIENTED_EDGE('',*,*,#24292,.F.);
#35420=ORIENTED_EDGE('',*,*,#24287,.F.);
#35421=ORIENTED_EDGE('',*,*,#24291,.F.);
#35422=ORIENTED_EDGE('',*,*,#24285,.F.);
#35423=ORIENTED_EDGE('',*,*,#24139,.F.);
#35424=ORIENTED_EDGE('',*,*,#24289,.F.);
#35425=ORIENTED_EDGE('',*,*,#24292,.T.);
#35426=ORIENTED_EDGE('',*,*,#24293,.F.);
#35427=ORIENTED_EDGE('',*,*,#24294,.T.);
#35428=ORIENTED_EDGE('',*,*,#24144,.T.);
#35429=ORIENTED_EDGE('',*,*,#24295,.T.);
#35430=ORIENTED_EDGE('',*,*,#24142,.T.);
#35431=ORIENTED_EDGE('',*,*,#24296,.F.);
#35432=ORIENTED_EDGE('',*,*,#24297,.T.);
#35433=ORIENTED_EDGE('',*,*,#24298,.T.);
#35434=ORIENTED_EDGE('',*,*,#24299,.T.);
#35435=ORIENTED_EDGE('',*,*,#24300,.T.);
#35436=ORIENTED_EDGE('',*,*,#24298,.F.);
#35437=ORIENTED_EDGE('',*,*,#24301,.T.);
#35438=ORIENTED_EDGE('',*,*,#24300,.F.);
#35439=ORIENTED_EDGE('',*,*,#24302,.F.);
#35440=ORIENTED_EDGE('',*,*,#24297,.F.);
#35441=ORIENTED_EDGE('',*,*,#24301,.F.);
#35442=ORIENTED_EDGE('',*,*,#24295,.F.);
#35443=ORIENTED_EDGE('',*,*,#24143,.F.);
#35444=ORIENTED_EDGE('',*,*,#24299,.F.);
#35445=ORIENTED_EDGE('',*,*,#24302,.T.);
#35446=ORIENTED_EDGE('',*,*,#24303,.F.);
#35447=ORIENTED_EDGE('',*,*,#24304,.T.);
#35448=ORIENTED_EDGE('',*,*,#24148,.T.);
#35449=ORIENTED_EDGE('',*,*,#24305,.T.);
#35450=ORIENTED_EDGE('',*,*,#24146,.T.);
#35451=ORIENTED_EDGE('',*,*,#24306,.F.);
#35452=ORIENTED_EDGE('',*,*,#24307,.T.);
#35453=ORIENTED_EDGE('',*,*,#24308,.T.);
#35454=ORIENTED_EDGE('',*,*,#24309,.T.);
#35455=ORIENTED_EDGE('',*,*,#24310,.T.);
#35456=ORIENTED_EDGE('',*,*,#24308,.F.);
#35457=ORIENTED_EDGE('',*,*,#24311,.T.);
#35458=ORIENTED_EDGE('',*,*,#24310,.F.);
#35459=ORIENTED_EDGE('',*,*,#24312,.F.);
#35460=ORIENTED_EDGE('',*,*,#24307,.F.);
#35461=ORIENTED_EDGE('',*,*,#24311,.F.);
#35462=ORIENTED_EDGE('',*,*,#24305,.F.);
#35463=ORIENTED_EDGE('',*,*,#24147,.F.);
#35464=ORIENTED_EDGE('',*,*,#24309,.F.);
#35465=ORIENTED_EDGE('',*,*,#24312,.T.);
#35466=ORIENTED_EDGE('',*,*,#24313,.F.);
#35467=ORIENTED_EDGE('',*,*,#24314,.T.);
#35468=ORIENTED_EDGE('',*,*,#24152,.T.);
#35469=ORIENTED_EDGE('',*,*,#24315,.T.);
#35470=ORIENTED_EDGE('',*,*,#24150,.T.);
#35471=ORIENTED_EDGE('',*,*,#24316,.F.);
#35472=ORIENTED_EDGE('',*,*,#24317,.T.);
#35473=ORIENTED_EDGE('',*,*,#24318,.T.);
#35474=ORIENTED_EDGE('',*,*,#24319,.T.);
#35475=ORIENTED_EDGE('',*,*,#24320,.T.);
#35476=ORIENTED_EDGE('',*,*,#24318,.F.);
#35477=ORIENTED_EDGE('',*,*,#24321,.T.);
#35478=ORIENTED_EDGE('',*,*,#24320,.F.);
#35479=ORIENTED_EDGE('',*,*,#24322,.F.);
#35480=ORIENTED_EDGE('',*,*,#24317,.F.);
#35481=ORIENTED_EDGE('',*,*,#24321,.F.);
#35482=ORIENTED_EDGE('',*,*,#24315,.F.);
#35483=ORIENTED_EDGE('',*,*,#24151,.F.);
#35484=ORIENTED_EDGE('',*,*,#24319,.F.);
#35485=ORIENTED_EDGE('',*,*,#24322,.T.);
#35486=ORIENTED_EDGE('',*,*,#24323,.F.);
#35487=ORIENTED_EDGE('',*,*,#24324,.T.);
#35488=ORIENTED_EDGE('',*,*,#24156,.T.);
#35489=ORIENTED_EDGE('',*,*,#24325,.T.);
#35490=ORIENTED_EDGE('',*,*,#24154,.T.);
#35491=ORIENTED_EDGE('',*,*,#24326,.F.);
#35492=ORIENTED_EDGE('',*,*,#24327,.T.);
#35493=ORIENTED_EDGE('',*,*,#24328,.T.);
#35494=ORIENTED_EDGE('',*,*,#24329,.T.);
#35495=ORIENTED_EDGE('',*,*,#24330,.T.);
#35496=ORIENTED_EDGE('',*,*,#24328,.F.);
#35497=ORIENTED_EDGE('',*,*,#24331,.T.);
#35498=ORIENTED_EDGE('',*,*,#24330,.F.);
#35499=ORIENTED_EDGE('',*,*,#24332,.F.);
#35500=ORIENTED_EDGE('',*,*,#24327,.F.);
#35501=ORIENTED_EDGE('',*,*,#24331,.F.);
#35502=ORIENTED_EDGE('',*,*,#24325,.F.);
#35503=ORIENTED_EDGE('',*,*,#24155,.F.);
#35504=ORIENTED_EDGE('',*,*,#24329,.F.);
#35505=ORIENTED_EDGE('',*,*,#24332,.T.);
#35506=ORIENTED_EDGE('',*,*,#24333,.F.);
#35507=ORIENTED_EDGE('',*,*,#24334,.T.);
#35508=ORIENTED_EDGE('',*,*,#24160,.T.);
#35509=ORIENTED_EDGE('',*,*,#24335,.T.);
#35510=ORIENTED_EDGE('',*,*,#24158,.T.);
#35511=ORIENTED_EDGE('',*,*,#24336,.F.);
#35512=ORIENTED_EDGE('',*,*,#24337,.T.);
#35513=ORIENTED_EDGE('',*,*,#24338,.T.);
#35514=ORIENTED_EDGE('',*,*,#24339,.T.);
#35515=ORIENTED_EDGE('',*,*,#24340,.T.);
#35516=ORIENTED_EDGE('',*,*,#24338,.F.);
#35517=ORIENTED_EDGE('',*,*,#24341,.T.);
#35518=ORIENTED_EDGE('',*,*,#24340,.F.);
#35519=ORIENTED_EDGE('',*,*,#24342,.F.);
#35520=ORIENTED_EDGE('',*,*,#24337,.F.);
#35521=ORIENTED_EDGE('',*,*,#24341,.F.);
#35522=ORIENTED_EDGE('',*,*,#24335,.F.);
#35523=ORIENTED_EDGE('',*,*,#24159,.F.);
#35524=ORIENTED_EDGE('',*,*,#24339,.F.);
#35525=ORIENTED_EDGE('',*,*,#24342,.T.);
#35526=ORIENTED_EDGE('',*,*,#24343,.F.);
#35527=ORIENTED_EDGE('',*,*,#24344,.T.);
#35528=ORIENTED_EDGE('',*,*,#24164,.T.);
#35529=ORIENTED_EDGE('',*,*,#24345,.T.);
#35530=ORIENTED_EDGE('',*,*,#24162,.T.);
#35531=ORIENTED_EDGE('',*,*,#24346,.F.);
#35532=ORIENTED_EDGE('',*,*,#24347,.T.);
#35533=ORIENTED_EDGE('',*,*,#24348,.T.);
#35534=ORIENTED_EDGE('',*,*,#24349,.T.);
#35535=ORIENTED_EDGE('',*,*,#24350,.T.);
#35536=ORIENTED_EDGE('',*,*,#24348,.F.);
#35537=ORIENTED_EDGE('',*,*,#24351,.T.);
#35538=ORIENTED_EDGE('',*,*,#24350,.F.);
#35539=ORIENTED_EDGE('',*,*,#24352,.F.);
#35540=ORIENTED_EDGE('',*,*,#24347,.F.);
#35541=ORIENTED_EDGE('',*,*,#24351,.F.);
#35542=ORIENTED_EDGE('',*,*,#24345,.F.);
#35543=ORIENTED_EDGE('',*,*,#24163,.F.);
#35544=ORIENTED_EDGE('',*,*,#24349,.F.);
#35545=ORIENTED_EDGE('',*,*,#24352,.T.);
#35546=ORIENTED_EDGE('',*,*,#24353,.F.);
#35547=ORIENTED_EDGE('',*,*,#24354,.T.);
#35548=ORIENTED_EDGE('',*,*,#24168,.T.);
#35549=ORIENTED_EDGE('',*,*,#24355,.T.);
#35550=ORIENTED_EDGE('',*,*,#24166,.T.);
#35551=ORIENTED_EDGE('',*,*,#24356,.F.);
#35552=ORIENTED_EDGE('',*,*,#24357,.T.);
#35553=ORIENTED_EDGE('',*,*,#24358,.T.);
#35554=ORIENTED_EDGE('',*,*,#24359,.T.);
#35555=ORIENTED_EDGE('',*,*,#24360,.T.);
#35556=ORIENTED_EDGE('',*,*,#24358,.F.);
#35557=ORIENTED_EDGE('',*,*,#24361,.T.);
#35558=ORIENTED_EDGE('',*,*,#24360,.F.);
#35559=ORIENTED_EDGE('',*,*,#24362,.F.);
#35560=ORIENTED_EDGE('',*,*,#24357,.F.);
#35561=ORIENTED_EDGE('',*,*,#24361,.F.);
#35562=ORIENTED_EDGE('',*,*,#24355,.F.);
#35563=ORIENTED_EDGE('',*,*,#24167,.F.);
#35564=ORIENTED_EDGE('',*,*,#24359,.F.);
#35565=ORIENTED_EDGE('',*,*,#24362,.T.);
#35566=ORIENTED_EDGE('',*,*,#24363,.F.);
#35567=ORIENTED_EDGE('',*,*,#24364,.T.);
#35568=ORIENTED_EDGE('',*,*,#24172,.T.);
#35569=ORIENTED_EDGE('',*,*,#24365,.T.);
#35570=ORIENTED_EDGE('',*,*,#24170,.T.);
#35571=ORIENTED_EDGE('',*,*,#24366,.F.);
#35572=ORIENTED_EDGE('',*,*,#24367,.T.);
#35573=ORIENTED_EDGE('',*,*,#24368,.T.);
#35574=ORIENTED_EDGE('',*,*,#24369,.T.);
#35575=ORIENTED_EDGE('',*,*,#24370,.T.);
#35576=ORIENTED_EDGE('',*,*,#24368,.F.);
#35577=ORIENTED_EDGE('',*,*,#24371,.T.);
#35578=ORIENTED_EDGE('',*,*,#24370,.F.);
#35579=ORIENTED_EDGE('',*,*,#24372,.F.);
#35580=ORIENTED_EDGE('',*,*,#24367,.F.);
#35581=ORIENTED_EDGE('',*,*,#24371,.F.);
#35582=ORIENTED_EDGE('',*,*,#24365,.F.);
#35583=ORIENTED_EDGE('',*,*,#24171,.F.);
#35584=ORIENTED_EDGE('',*,*,#24369,.F.);
#35585=ORIENTED_EDGE('',*,*,#24372,.T.);
#35586=ORIENTED_EDGE('',*,*,#24373,.F.);
#35587=ORIENTED_EDGE('',*,*,#24374,.T.);
#35588=ORIENTED_EDGE('',*,*,#24176,.T.);
#35589=ORIENTED_EDGE('',*,*,#24375,.T.);
#35590=ORIENTED_EDGE('',*,*,#24174,.T.);
#35591=ORIENTED_EDGE('',*,*,#24376,.F.);
#35592=ORIENTED_EDGE('',*,*,#24377,.T.);
#35593=ORIENTED_EDGE('',*,*,#24378,.T.);
#35594=ORIENTED_EDGE('',*,*,#24379,.T.);
#35595=ORIENTED_EDGE('',*,*,#24380,.T.);
#35596=ORIENTED_EDGE('',*,*,#24378,.F.);
#35597=ORIENTED_EDGE('',*,*,#24381,.T.);
#35598=ORIENTED_EDGE('',*,*,#24380,.F.);
#35599=ORIENTED_EDGE('',*,*,#24382,.F.);
#35600=ORIENTED_EDGE('',*,*,#24377,.F.);
#35601=ORIENTED_EDGE('',*,*,#24381,.F.);
#35602=ORIENTED_EDGE('',*,*,#24375,.F.);
#35603=ORIENTED_EDGE('',*,*,#24175,.F.);
#35604=ORIENTED_EDGE('',*,*,#24379,.F.);
#35605=ORIENTED_EDGE('',*,*,#24382,.T.);
#35606=ORIENTED_EDGE('',*,*,#24383,.F.);
#35607=ORIENTED_EDGE('',*,*,#24384,.T.);
#35608=ORIENTED_EDGE('',*,*,#24180,.T.);
#35609=ORIENTED_EDGE('',*,*,#24385,.T.);
#35610=ORIENTED_EDGE('',*,*,#24178,.T.);
#35611=ORIENTED_EDGE('',*,*,#24386,.F.);
#35612=ORIENTED_EDGE('',*,*,#24387,.T.);
#35613=ORIENTED_EDGE('',*,*,#24388,.T.);
#35614=ORIENTED_EDGE('',*,*,#24389,.T.);
#35615=ORIENTED_EDGE('',*,*,#24390,.T.);
#35616=ORIENTED_EDGE('',*,*,#24388,.F.);
#35617=ORIENTED_EDGE('',*,*,#24391,.T.);
#35618=ORIENTED_EDGE('',*,*,#24390,.F.);
#35619=ORIENTED_EDGE('',*,*,#24392,.F.);
#35620=ORIENTED_EDGE('',*,*,#24387,.F.);
#35621=ORIENTED_EDGE('',*,*,#24391,.F.);
#35622=ORIENTED_EDGE('',*,*,#24385,.F.);
#35623=ORIENTED_EDGE('',*,*,#24179,.F.);
#35624=ORIENTED_EDGE('',*,*,#24389,.F.);
#35625=ORIENTED_EDGE('',*,*,#24392,.T.);
#35626=ORIENTED_EDGE('',*,*,#24393,.F.);
#35627=ORIENTED_EDGE('',*,*,#24394,.T.);
#35628=ORIENTED_EDGE('',*,*,#24184,.T.);
#35629=ORIENTED_EDGE('',*,*,#24395,.T.);
#35630=ORIENTED_EDGE('',*,*,#24182,.T.);
#35631=ORIENTED_EDGE('',*,*,#24396,.F.);
#35632=ORIENTED_EDGE('',*,*,#24397,.T.);
#35633=ORIENTED_EDGE('',*,*,#24398,.T.);
#35634=ORIENTED_EDGE('',*,*,#24399,.T.);
#35635=ORIENTED_EDGE('',*,*,#24400,.T.);
#35636=ORIENTED_EDGE('',*,*,#24398,.F.);
#35637=ORIENTED_EDGE('',*,*,#24401,.T.);
#35638=ORIENTED_EDGE('',*,*,#24400,.F.);
#35639=ORIENTED_EDGE('',*,*,#24402,.F.);
#35640=ORIENTED_EDGE('',*,*,#24397,.F.);
#35641=ORIENTED_EDGE('',*,*,#24401,.F.);
#35642=ORIENTED_EDGE('',*,*,#24395,.F.);
#35643=ORIENTED_EDGE('',*,*,#24183,.F.);
#35644=ORIENTED_EDGE('',*,*,#24399,.F.);
#35645=ORIENTED_EDGE('',*,*,#24402,.T.);
#35646=ORIENTED_EDGE('',*,*,#24403,.F.);
#35647=ORIENTED_EDGE('',*,*,#24404,.T.);
#35648=ORIENTED_EDGE('',*,*,#24188,.T.);
#35649=ORIENTED_EDGE('',*,*,#24405,.T.);
#35650=ORIENTED_EDGE('',*,*,#24186,.T.);
#35651=ORIENTED_EDGE('',*,*,#24406,.F.);
#35652=ORIENTED_EDGE('',*,*,#24407,.T.);
#35653=ORIENTED_EDGE('',*,*,#24408,.T.);
#35654=ORIENTED_EDGE('',*,*,#24409,.T.);
#35655=ORIENTED_EDGE('',*,*,#24410,.T.);
#35656=ORIENTED_EDGE('',*,*,#24408,.F.);
#35657=ORIENTED_EDGE('',*,*,#24411,.T.);
#35658=ORIENTED_EDGE('',*,*,#24410,.F.);
#35659=ORIENTED_EDGE('',*,*,#24412,.F.);
#35660=ORIENTED_EDGE('',*,*,#24407,.F.);
#35661=ORIENTED_EDGE('',*,*,#24411,.F.);
#35662=ORIENTED_EDGE('',*,*,#24405,.F.);
#35663=ORIENTED_EDGE('',*,*,#24187,.F.);
#35664=ORIENTED_EDGE('',*,*,#24409,.F.);
#35665=ORIENTED_EDGE('',*,*,#24412,.T.);
#35666=ORIENTED_EDGE('',*,*,#24413,.F.);
#35667=ORIENTED_EDGE('',*,*,#24414,.T.);
#35668=ORIENTED_EDGE('',*,*,#24192,.T.);
#35669=ORIENTED_EDGE('',*,*,#24415,.T.);
#35670=ORIENTED_EDGE('',*,*,#24190,.T.);
#35671=ORIENTED_EDGE('',*,*,#24416,.F.);
#35672=ORIENTED_EDGE('',*,*,#24417,.T.);
#35673=ORIENTED_EDGE('',*,*,#24418,.T.);
#35674=ORIENTED_EDGE('',*,*,#24419,.T.);
#35675=ORIENTED_EDGE('',*,*,#24420,.T.);
#35676=ORIENTED_EDGE('',*,*,#24418,.F.);
#35677=ORIENTED_EDGE('',*,*,#24421,.T.);
#35678=ORIENTED_EDGE('',*,*,#24420,.F.);
#35679=ORIENTED_EDGE('',*,*,#24422,.F.);
#35680=ORIENTED_EDGE('',*,*,#24417,.F.);
#35681=ORIENTED_EDGE('',*,*,#24421,.F.);
#35682=ORIENTED_EDGE('',*,*,#24415,.F.);
#35683=ORIENTED_EDGE('',*,*,#24191,.F.);
#35684=ORIENTED_EDGE('',*,*,#24419,.F.);
#35685=ORIENTED_EDGE('',*,*,#24422,.T.);
#35686=ORIENTED_EDGE('',*,*,#24423,.F.);
#35687=ORIENTED_EDGE('',*,*,#24424,.T.);
#35688=ORIENTED_EDGE('',*,*,#24196,.T.);
#35689=ORIENTED_EDGE('',*,*,#24425,.T.);
#35690=ORIENTED_EDGE('',*,*,#24194,.T.);
#35691=ORIENTED_EDGE('',*,*,#24426,.F.);
#35692=ORIENTED_EDGE('',*,*,#24427,.T.);
#35693=ORIENTED_EDGE('',*,*,#24428,.T.);
#35694=ORIENTED_EDGE('',*,*,#24429,.T.);
#35695=ORIENTED_EDGE('',*,*,#24430,.T.);
#35696=ORIENTED_EDGE('',*,*,#24428,.F.);
#35697=ORIENTED_EDGE('',*,*,#24431,.T.);
#35698=ORIENTED_EDGE('',*,*,#24430,.F.);
#35699=ORIENTED_EDGE('',*,*,#24432,.F.);
#35700=ORIENTED_EDGE('',*,*,#24427,.F.);
#35701=ORIENTED_EDGE('',*,*,#24431,.F.);
#35702=ORIENTED_EDGE('',*,*,#24425,.F.);
#35703=ORIENTED_EDGE('',*,*,#24195,.F.);
#35704=ORIENTED_EDGE('',*,*,#24429,.F.);
#35705=ORIENTED_EDGE('',*,*,#24432,.T.);
#35706=ORIENTED_EDGE('',*,*,#24433,.F.);
#35707=ORIENTED_EDGE('',*,*,#24434,.T.);
#35708=ORIENTED_EDGE('',*,*,#24200,.T.);
#35709=ORIENTED_EDGE('',*,*,#24435,.T.);
#35710=ORIENTED_EDGE('',*,*,#24198,.T.);
#35711=ORIENTED_EDGE('',*,*,#24436,.F.);
#35712=ORIENTED_EDGE('',*,*,#24437,.T.);
#35713=ORIENTED_EDGE('',*,*,#24438,.T.);
#35714=ORIENTED_EDGE('',*,*,#24439,.T.);
#35715=ORIENTED_EDGE('',*,*,#24440,.T.);
#35716=ORIENTED_EDGE('',*,*,#24438,.F.);
#35717=ORIENTED_EDGE('',*,*,#24441,.T.);
#35718=ORIENTED_EDGE('',*,*,#24440,.F.);
#35719=ORIENTED_EDGE('',*,*,#24442,.F.);
#35720=ORIENTED_EDGE('',*,*,#24437,.F.);
#35721=ORIENTED_EDGE('',*,*,#24441,.F.);
#35722=ORIENTED_EDGE('',*,*,#24435,.F.);
#35723=ORIENTED_EDGE('',*,*,#24199,.F.);
#35724=ORIENTED_EDGE('',*,*,#24439,.F.);
#35725=ORIENTED_EDGE('',*,*,#24442,.T.);
#35726=ORIENTED_EDGE('',*,*,#24443,.F.);
#35727=ORIENTED_EDGE('',*,*,#24444,.T.);
#35728=ORIENTED_EDGE('',*,*,#24208,.T.);
#35729=ORIENTED_EDGE('',*,*,#24445,.T.);
#35730=ORIENTED_EDGE('',*,*,#24206,.T.);
#35731=ORIENTED_EDGE('',*,*,#24446,.F.);
#35732=ORIENTED_EDGE('',*,*,#24447,.T.);
#35733=ORIENTED_EDGE('',*,*,#24448,.T.);
#35734=ORIENTED_EDGE('',*,*,#24449,.T.);
#35735=ORIENTED_EDGE('',*,*,#24450,.T.);
#35736=ORIENTED_EDGE('',*,*,#24445,.F.);
#35737=ORIENTED_EDGE('',*,*,#24207,.F.);
#35738=ORIENTED_EDGE('',*,*,#24448,.F.);
#35739=ORIENTED_EDGE('',*,*,#24451,.T.);
#35740=ORIENTED_EDGE('',*,*,#24450,.F.);
#35741=ORIENTED_EDGE('',*,*,#24452,.F.);
#35742=ORIENTED_EDGE('',*,*,#24447,.F.);
#35743=ORIENTED_EDGE('',*,*,#24451,.F.);
#35744=ORIENTED_EDGE('',*,*,#24453,.F.);
#35745=ORIENTED_EDGE('',*,*,#24454,.T.);
#35746=ORIENTED_EDGE('',*,*,#24204,.T.);
#35747=ORIENTED_EDGE('',*,*,#24455,.T.);
#35748=ORIENTED_EDGE('',*,*,#24202,.T.);
#35749=ORIENTED_EDGE('',*,*,#24456,.F.);
#35750=ORIENTED_EDGE('',*,*,#24457,.T.);
#35751=ORIENTED_EDGE('',*,*,#24458,.T.);
#35752=ORIENTED_EDGE('',*,*,#24459,.T.);
#35753=ORIENTED_EDGE('',*,*,#24460,.T.);
#35754=ORIENTED_EDGE('',*,*,#24458,.F.);
#35755=ORIENTED_EDGE('',*,*,#24461,.T.);
#35756=ORIENTED_EDGE('',*,*,#24460,.F.);
#35757=ORIENTED_EDGE('',*,*,#24462,.F.);
#35758=ORIENTED_EDGE('',*,*,#24457,.F.);
#35759=ORIENTED_EDGE('',*,*,#24461,.F.);
#35760=ORIENTED_EDGE('',*,*,#24463,.T.);
#35761=ORIENTED_EDGE('',*,*,#24464,.T.);
#35762=ORIENTED_EDGE('',*,*,#24465,.T.);
#35763=ORIENTED_EDGE('',*,*,#24466,.T.);
#35764=ORIENTED_EDGE('',*,*,#24464,.F.);
#35765=ORIENTED_EDGE('',*,*,#24467,.T.);
#35766=ORIENTED_EDGE('',*,*,#24212,.F.);
#35767=ORIENTED_EDGE('',*,*,#24468,.F.);
#35768=ORIENTED_EDGE('',*,*,#24106,.F.);
#35769=ORIENTED_EDGE('',*,*,#24105,.T.);
#35770=ORIENTED_EDGE('',*,*,#24469,.T.);
#35771=ORIENTED_EDGE('',*,*,#24210,.T.);
#35772=ORIENTED_EDGE('',*,*,#24467,.F.);
#35773=ORIENTED_EDGE('',*,*,#24463,.F.);
#35774=ORIENTED_EDGE('',*,*,#24470,.T.);
#35775=ORIENTED_EDGE('',*,*,#24443,.T.);
#35776=ORIENTED_EDGE('',*,*,#24471,.T.);
#35777=ORIENTED_EDGE('',*,*,#24453,.T.);
#35778=ORIENTED_EDGE('',*,*,#24472,.T.);
#35779=ORIENTED_EDGE('',*,*,#24433,.T.);
#35780=ORIENTED_EDGE('',*,*,#24473,.T.);
#35781=ORIENTED_EDGE('',*,*,#24423,.T.);
#35782=ORIENTED_EDGE('',*,*,#24474,.T.);
#35783=ORIENTED_EDGE('',*,*,#24413,.T.);
#35784=ORIENTED_EDGE('',*,*,#24475,.T.);
#35785=ORIENTED_EDGE('',*,*,#24403,.T.);
#35786=ORIENTED_EDGE('',*,*,#24476,.T.);
#35787=ORIENTED_EDGE('',*,*,#24393,.T.);
#35788=ORIENTED_EDGE('',*,*,#24477,.T.);
#35789=ORIENTED_EDGE('',*,*,#24383,.T.);
#35790=ORIENTED_EDGE('',*,*,#24478,.T.);
#35791=ORIENTED_EDGE('',*,*,#24373,.T.);
#35792=ORIENTED_EDGE('',*,*,#24479,.T.);
#35793=ORIENTED_EDGE('',*,*,#24363,.T.);
#35794=ORIENTED_EDGE('',*,*,#24480,.T.);
#35795=ORIENTED_EDGE('',*,*,#24353,.T.);
#35796=ORIENTED_EDGE('',*,*,#24481,.T.);
#35797=ORIENTED_EDGE('',*,*,#24343,.T.);
#35798=ORIENTED_EDGE('',*,*,#24482,.T.);
#35799=ORIENTED_EDGE('',*,*,#24333,.T.);
#35800=ORIENTED_EDGE('',*,*,#24483,.T.);
#35801=ORIENTED_EDGE('',*,*,#24323,.T.);
#35802=ORIENTED_EDGE('',*,*,#24484,.T.);
#35803=ORIENTED_EDGE('',*,*,#24313,.T.);
#35804=ORIENTED_EDGE('',*,*,#24485,.T.);
#35805=ORIENTED_EDGE('',*,*,#24303,.T.);
#35806=ORIENTED_EDGE('',*,*,#24486,.T.);
#35807=ORIENTED_EDGE('',*,*,#24293,.T.);
#35808=ORIENTED_EDGE('',*,*,#24487,.T.);
#35809=ORIENTED_EDGE('',*,*,#24283,.T.);
#35810=ORIENTED_EDGE('',*,*,#24488,.T.);
#35811=ORIENTED_EDGE('',*,*,#24273,.T.);
#35812=ORIENTED_EDGE('',*,*,#24489,.T.);
#35813=ORIENTED_EDGE('',*,*,#24263,.T.);
#35814=ORIENTED_EDGE('',*,*,#24490,.T.);
#35815=ORIENTED_EDGE('',*,*,#24253,.T.);
#35816=ORIENTED_EDGE('',*,*,#24491,.T.);
#35817=ORIENTED_EDGE('',*,*,#24243,.T.);
#35818=ORIENTED_EDGE('',*,*,#24492,.T.);
#35819=ORIENTED_EDGE('',*,*,#24233,.T.);
#35820=ORIENTED_EDGE('',*,*,#24493,.T.);
#35821=ORIENTED_EDGE('',*,*,#24223,.T.);
#35822=ORIENTED_EDGE('',*,*,#24494,.T.);
#35823=ORIENTED_EDGE('',*,*,#24213,.T.);
#35824=ORIENTED_EDGE('',*,*,#24495,.T.);
#35825=ORIENTED_EDGE('',*,*,#24095,.F.);
#35826=ORIENTED_EDGE('',*,*,#24466,.F.);
#35827=ORIENTED_EDGE('',*,*,#24496,.T.);
#35828=ORIENTED_EDGE('',*,*,#23948,.T.);
#35829=ORIENTED_EDGE('',*,*,#24496,.F.);
#35830=ORIENTED_EDGE('',*,*,#24465,.F.);
#35831=ORIENTED_EDGE('',*,*,#24455,.F.);
#35832=ORIENTED_EDGE('',*,*,#24203,.F.);
#35833=ORIENTED_EDGE('',*,*,#24205,.F.);
#35834=ORIENTED_EDGE('',*,*,#24454,.F.);
#35835=ORIENTED_EDGE('',*,*,#24471,.F.);
#35836=ORIENTED_EDGE('',*,*,#24446,.T.);
#35837=ORIENTED_EDGE('',*,*,#24459,.F.);
#35838=ORIENTED_EDGE('',*,*,#24462,.T.);
#35839=ORIENTED_EDGE('',*,*,#24201,.F.);
#35840=ORIENTED_EDGE('',*,*,#24434,.F.);
#35841=ORIENTED_EDGE('',*,*,#24472,.F.);
#35842=ORIENTED_EDGE('',*,*,#24456,.T.);
#35843=ORIENTED_EDGE('',*,*,#24197,.F.);
#35844=ORIENTED_EDGE('',*,*,#24424,.F.);
#35845=ORIENTED_EDGE('',*,*,#24473,.F.);
#35846=ORIENTED_EDGE('',*,*,#24436,.T.);
#35847=ORIENTED_EDGE('',*,*,#24193,.F.);
#35848=ORIENTED_EDGE('',*,*,#24414,.F.);
#35849=ORIENTED_EDGE('',*,*,#24474,.F.);
#35850=ORIENTED_EDGE('',*,*,#24426,.T.);
#35851=ORIENTED_EDGE('',*,*,#24189,.F.);
#35852=ORIENTED_EDGE('',*,*,#24404,.F.);
#35853=ORIENTED_EDGE('',*,*,#24475,.F.);
#35854=ORIENTED_EDGE('',*,*,#24416,.T.);
#35855=ORIENTED_EDGE('',*,*,#24185,.F.);
#35856=ORIENTED_EDGE('',*,*,#24394,.F.);
#35857=ORIENTED_EDGE('',*,*,#24476,.F.);
#35858=ORIENTED_EDGE('',*,*,#24406,.T.);
#35859=ORIENTED_EDGE('',*,*,#24181,.F.);
#35860=ORIENTED_EDGE('',*,*,#24384,.F.);
#35861=ORIENTED_EDGE('',*,*,#24477,.F.);
#35862=ORIENTED_EDGE('',*,*,#24396,.T.);
#35863=ORIENTED_EDGE('',*,*,#24177,.F.);
#35864=ORIENTED_EDGE('',*,*,#24374,.F.);
#35865=ORIENTED_EDGE('',*,*,#24478,.F.);
#35866=ORIENTED_EDGE('',*,*,#24386,.T.);
#35867=ORIENTED_EDGE('',*,*,#24173,.F.);
#35868=ORIENTED_EDGE('',*,*,#24364,.F.);
#35869=ORIENTED_EDGE('',*,*,#24479,.F.);
#35870=ORIENTED_EDGE('',*,*,#24376,.T.);
#35871=ORIENTED_EDGE('',*,*,#24169,.F.);
#35872=ORIENTED_EDGE('',*,*,#24354,.F.);
#35873=ORIENTED_EDGE('',*,*,#24480,.F.);
#35874=ORIENTED_EDGE('',*,*,#24366,.T.);
#35875=ORIENTED_EDGE('',*,*,#24165,.F.);
#35876=ORIENTED_EDGE('',*,*,#24344,.F.);
#35877=ORIENTED_EDGE('',*,*,#24481,.F.);
#35878=ORIENTED_EDGE('',*,*,#24356,.T.);
#35879=ORIENTED_EDGE('',*,*,#24161,.F.);
#35880=ORIENTED_EDGE('',*,*,#24334,.F.);
#35881=ORIENTED_EDGE('',*,*,#24482,.F.);
#35882=ORIENTED_EDGE('',*,*,#24346,.T.);
#35883=ORIENTED_EDGE('',*,*,#24157,.F.);
#35884=ORIENTED_EDGE('',*,*,#24324,.F.);
#35885=ORIENTED_EDGE('',*,*,#24483,.F.);
#35886=ORIENTED_EDGE('',*,*,#24336,.T.);
#35887=ORIENTED_EDGE('',*,*,#24153,.F.);
#35888=ORIENTED_EDGE('',*,*,#24314,.F.);
#35889=ORIENTED_EDGE('',*,*,#24484,.F.);
#35890=ORIENTED_EDGE('',*,*,#24326,.T.);
#35891=ORIENTED_EDGE('',*,*,#24149,.F.);
#35892=ORIENTED_EDGE('',*,*,#24304,.F.);
#35893=ORIENTED_EDGE('',*,*,#24485,.F.);
#35894=ORIENTED_EDGE('',*,*,#24316,.T.);
#35895=ORIENTED_EDGE('',*,*,#24145,.F.);
#35896=ORIENTED_EDGE('',*,*,#24294,.F.);
#35897=ORIENTED_EDGE('',*,*,#24486,.F.);
#35898=ORIENTED_EDGE('',*,*,#24306,.T.);
#35899=ORIENTED_EDGE('',*,*,#24141,.F.);
#35900=ORIENTED_EDGE('',*,*,#24284,.F.);
#35901=ORIENTED_EDGE('',*,*,#24487,.F.);
#35902=ORIENTED_EDGE('',*,*,#24296,.T.);
#35903=ORIENTED_EDGE('',*,*,#24137,.F.);
#35904=ORIENTED_EDGE('',*,*,#24274,.F.);
#35905=ORIENTED_EDGE('',*,*,#24488,.F.);
#35906=ORIENTED_EDGE('',*,*,#24286,.T.);
#35907=ORIENTED_EDGE('',*,*,#24133,.F.);
#35908=ORIENTED_EDGE('',*,*,#24264,.F.);
#35909=ORIENTED_EDGE('',*,*,#24489,.F.);
#35910=ORIENTED_EDGE('',*,*,#24276,.T.);
#35911=ORIENTED_EDGE('',*,*,#24129,.F.);
#35912=ORIENTED_EDGE('',*,*,#24254,.F.);
#35913=ORIENTED_EDGE('',*,*,#24490,.F.);
#35914=ORIENTED_EDGE('',*,*,#24266,.T.);
#35915=ORIENTED_EDGE('',*,*,#24125,.F.);
#35916=ORIENTED_EDGE('',*,*,#24244,.F.);
#35917=ORIENTED_EDGE('',*,*,#24491,.F.);
#35918=ORIENTED_EDGE('',*,*,#24256,.T.);
#35919=ORIENTED_EDGE('',*,*,#24121,.F.);
#35920=ORIENTED_EDGE('',*,*,#24234,.F.);
#35921=ORIENTED_EDGE('',*,*,#24492,.F.);
#35922=ORIENTED_EDGE('',*,*,#24246,.T.);
#35923=ORIENTED_EDGE('',*,*,#24117,.F.);
#35924=ORIENTED_EDGE('',*,*,#24224,.F.);
#35925=ORIENTED_EDGE('',*,*,#24493,.F.);
#35926=ORIENTED_EDGE('',*,*,#24236,.T.);
#35927=ORIENTED_EDGE('',*,*,#24113,.F.);
#35928=ORIENTED_EDGE('',*,*,#24214,.F.);
#35929=ORIENTED_EDGE('',*,*,#24494,.F.);
#35930=ORIENTED_EDGE('',*,*,#24226,.T.);
#35931=ORIENTED_EDGE('',*,*,#24109,.F.);
#35932=ORIENTED_EDGE('',*,*,#24096,.F.);
#35933=ORIENTED_EDGE('',*,*,#24495,.F.);
#35934=ORIENTED_EDGE('',*,*,#24216,.T.);
#35935=ORIENTED_EDGE('',*,*,#24469,.F.);
#35936=ORIENTED_EDGE('',*,*,#24107,.F.);
#35937=ORIENTED_EDGE('',*,*,#24468,.T.);
#35938=ORIENTED_EDGE('',*,*,#24211,.F.);
#35939=ORIENTED_EDGE('',*,*,#24209,.F.);
#35940=ORIENTED_EDGE('',*,*,#24444,.F.);
#35941=ORIENTED_EDGE('',*,*,#24470,.F.);
#35942=ORIENTED_EDGE('',*,*,#24094,.T.);
#35943=ORIENTED_EDGE('',*,*,#24089,.F.);
#35944=ORIENTED_EDGE('',*,*,#24092,.F.);
#35945=ORIENTED_EDGE('',*,*,#24071,.F.);
#35946=ORIENTED_EDGE('',*,*,#24074,.F.);
#35947=ORIENTED_EDGE('',*,*,#24497,.F.);
#35948=ORIENTED_EDGE('',*,*,#23985,.F.);
#35949=ORIENTED_EDGE('',*,*,#23999,.F.);
#35950=ORIENTED_EDGE('',*,*,#24013,.F.);
#35951=ORIENTED_EDGE('',*,*,#24017,.F.);
#35952=ORIENTED_EDGE('',*,*,#24044,.F.);
#35953=ORIENTED_EDGE('',*,*,#24050,.F.);
#35954=ORIENTED_EDGE('',*,*,#24051,.F.);
#35955=ORIENTED_EDGE('',*,*,#24040,.F.);
#35956=ORIENTED_EDGE('',*,*,#24035,.F.);
#35957=ORIENTED_EDGE('',*,*,#24009,.F.);
#35958=ORIENTED_EDGE('',*,*,#23994,.F.);
#35959=ORIENTED_EDGE('',*,*,#23986,.F.);
#35960=ORIENTED_EDGE('',*,*,#24497,.T.);
#35961=ORIENTED_EDGE('',*,*,#23993,.F.);
#35962=ORIENTED_EDGE('',*,*,#23988,.F.);
#35963=ORIENTED_EDGE('',*,*,#23960,.F.);
#35964=ORIENTED_EDGE('',*,*,#24498,.T.);
#35965=ORIENTED_EDGE('',*,*,#24053,.T.);
#35966=ORIENTED_EDGE('',*,*,#24075,.T.);
#35967=ORIENTED_EDGE('',*,*,#24069,.T.);
#35968=ORIENTED_EDGE('',*,*,#24077,.T.);
#35969=ORIENTED_EDGE('',*,*,#24087,.T.);
#35970=ORIENTED_EDGE('',*,*,#24055,.T.);
#35971=ORIENTED_EDGE('',*,*,#24054,.T.);
#35972=ORIENTED_EDGE('',*,*,#24498,.F.);
#35973=ORIENTED_EDGE('',*,*,#24449,.F.);
#35974=ORIENTED_EDGE('',*,*,#24452,.T.);
#37785=CYLINDRICAL_SURFACE('',#44277,17.);
#37786=CYLINDRICAL_SURFACE('',#44286,19.);
#37787=CYLINDRICAL_SURFACE('',#44303,41.);
#37788=CYLINDRICAL_SURFACE('',#44321,1.);
#37789=CYLINDRICAL_SURFACE('',#44331,1.);
#37790=CYLINDRICAL_SURFACE('',#44336,18.);
#37791=CYLINDRICAL_SURFACE('',#44351,18.);
#37792=CYLINDRICAL_SURFACE('',#44353,1.);
#37793=CYLINDRICAL_SURFACE('',#44358,15.5);
#37794=CYLINDRICAL_SURFACE('',#44365,1.);
#37795=CYLINDRICAL_SURFACE('',#44367,1.);
#37796=CYLINDRICAL_SURFACE('',#44368,1.);
#37797=CYLINDRICAL_SURFACE('',#44376,15.5);
#37798=CYLINDRICAL_SURFACE('',#44378,1.);
#37799=CYLINDRICAL_SURFACE('',#44388,18.);
#37800=CYLINDRICAL_SURFACE('',#44390,1.);
#37801=CYLINDRICAL_SURFACE('',#44397,39.);
#37802=CYLINDRICAL_SURFACE('',#44404,1.);
#37803=CYLINDRICAL_SURFACE('',#44405,1.);
#37804=CYLINDRICAL_SURFACE('',#44411,39.);
#37805=CYLINDRICAL_SURFACE('',#44413,39.);
#37806=CYLINDRICAL_SURFACE('',#44417,1.);
#37807=CYLINDRICAL_SURFACE('',#44418,1.);
#37808=CYLINDRICAL_SURFACE('',#44424,0.999999999999999);
#37809=CYLINDRICAL_SURFACE('',#44430,12.);
#37810=CYLINDRICAL_SURFACE('',#44513,0.999999999999999);
#37811=CYLINDRICAL_SURFACE('',#44516,1.);
#37812=CYLINDRICAL_SURFACE('',#44520,12.);
#37813=CYLINDRICAL_SURFACE('',#44526,1.);
#37814=CYLINDRICAL_SURFACE('',#44530,12.);
#37815=CYLINDRICAL_SURFACE('',#44536,0.999999999999999);
#37816=CYLINDRICAL_SURFACE('',#44540,12.);
#37817=CYLINDRICAL_SURFACE('',#44546,1.);
#37818=CYLINDRICAL_SURFACE('',#44550,12.);
#37819=CYLINDRICAL_SURFACE('',#44556,1.);
#37820=CYLINDRICAL_SURFACE('',#44560,12.);
#37821=CYLINDRICAL_SURFACE('',#44566,1.);
#37822=CYLINDRICAL_SURFACE('',#44570,12.);
#37823=CYLINDRICAL_SURFACE('',#44576,1.);
#37824=CYLINDRICAL_SURFACE('',#44580,12.);
#37825=CYLINDRICAL_SURFACE('',#44586,0.999999999999999);
#37826=CYLINDRICAL_SURFACE('',#44590,12.);
#37827=CYLINDRICAL_SURFACE('',#44596,1.);
#37828=CYLINDRICAL_SURFACE('',#44600,12.);
#37829=CYLINDRICAL_SURFACE('',#44606,1.);
#37830=CYLINDRICAL_SURFACE('',#44610,12.);
#37831=CYLINDRICAL_SURFACE('',#44616,1.);
#37832=CYLINDRICAL_SURFACE('',#44620,12.);
#37833=CYLINDRICAL_SURFACE('',#44626,0.999999999999999);
#37834=CYLINDRICAL_SURFACE('',#44630,12.);
#37835=CYLINDRICAL_SURFACE('',#44636,0.999999999999999);
#37836=CYLINDRICAL_SURFACE('',#44640,12.);
#37837=CYLINDRICAL_SURFACE('',#44646,0.999999999999999);
#37838=CYLINDRICAL_SURFACE('',#44650,12.);
#37839=CYLINDRICAL_SURFACE('',#44656,1.);
#37840=CYLINDRICAL_SURFACE('',#44660,12.);
#37841=CYLINDRICAL_SURFACE('',#44666,1.);
#37842=CYLINDRICAL_SURFACE('',#44670,12.);
#37843=CYLINDRICAL_SURFACE('',#44676,1.);
#37844=CYLINDRICAL_SURFACE('',#44680,12.);
#37845=CYLINDRICAL_SURFACE('',#44686,1.);
#37846=CYLINDRICAL_SURFACE('',#44690,12.);
#37847=CYLINDRICAL_SURFACE('',#44696,1.);
#37848=CYLINDRICAL_SURFACE('',#44700,12.);
#37849=CYLINDRICAL_SURFACE('',#44706,1.);
#37850=CYLINDRICAL_SURFACE('',#44710,12.);
#37851=CYLINDRICAL_SURFACE('',#44716,1.);
#37852=CYLINDRICAL_SURFACE('',#44720,12.);
#37853=CYLINDRICAL_SURFACE('',#44726,1.);
#37854=CYLINDRICAL_SURFACE('',#44730,12.);
#37855=CYLINDRICAL_SURFACE('',#44736,1.);
#37856=CYLINDRICAL_SURFACE('',#44740,12.);
#37857=CYLINDRICAL_SURFACE('',#44746,1.);
#37858=CYLINDRICAL_SURFACE('',#44751,12.);
#37859=CYLINDRICAL_SURFACE('',#44755,1.);
#37860=CYLINDRICAL_SURFACE('',#44759,12.);
#37861=CYLINDRICAL_SURFACE('',#44772,13.8);
#37862=CYLINDRICAL_SURFACE('',#44800,12.9);
#37863=CYLINDRICAL_SURFACE('',#44806,15.5);
#39891=ADVANCED_FACE('',(#4088),#991,.T.);
#39892=ADVANCED_FACE('',(#4089),#37785,.T.);
#39893=ADVANCED_FACE('',(#4090,#1077),#1641,.T.);
#39894=ADVANCED_FACE('',(#4091),#992,.T.);
#39895=ADVANCED_FACE('',(#4092),#37786,.T.);
#39896=ADVANCED_FACE('',(#4093,#1078),#1642,.T.);
#39897=ADVANCED_FACE('',(#4094),#993,.T.);
#39898=ADVANCED_FACE('',(#4095),#745,.T.);
#39899=ADVANCED_FACE('',(#4096,#1079),#1643,.T.);
#39900=ADVANCED_FACE('',(#4097),#994,.T.);
#39901=ADVANCED_FACE('',(#4098),#37787,.T.);
#39902=ADVANCED_FACE('',(#4099),#746,.T.);
#39903=ADVANCED_FACE('',(#4100),#995,.T.);
#39904=ADVANCED_FACE('',(#4101),#747,.T.);
#39905=ADVANCED_FACE('',(#4102),#37788,.T.);
#39906=ADVANCED_FACE('',(#4103),#996,.T.);
#39907=ADVANCED_FACE('',(#4104),#567,.T.);
#39908=ADVANCED_FACE('',(#4105),#37789,.T.);
#39909=ADVANCED_FACE('',(#4106),#568,.T.);
#39910=ADVANCED_FACE('',(#4107),#37790,.F.);
#39911=ADVANCED_FACE('',(#4108),#997,.T.);
#39912=ADVANCED_FACE('',(#4109,#1080),#1644,.T.);
#39913=ADVANCED_FACE('',(#4110),#998,.T.);
#39914=ADVANCED_FACE('',(#4111),#37791,.F.);
#39915=ADVANCED_FACE('',(#4112),#37792,.T.);
#39916=ADVANCED_FACE('',(#4113),#569,.T.);
#39917=ADVANCED_FACE('',(#4114),#37793,.F.);
#39918=ADVANCED_FACE('',(#4115),#999,.T.);
#39919=ADVANCED_FACE('',(#4116),#1000,.T.);
#39920=ADVANCED_FACE('',(#4117),#37794,.T.);
#39921=ADVANCED_FACE('',(#4118),#1645,.F.);
#39922=ADVANCED_FACE('',(#4119),#37795,.T.);
#39923=ADVANCED_FACE('',(#4120),#37796,.T.);
#39924=ADVANCED_FACE('',(#4121),#570,.T.);
#39925=ADVANCED_FACE('',(#4122),#1001,.T.);
#39926=ADVANCED_FACE('',(#4123),#37797,.F.);
#39927=ADVANCED_FACE('',(#4124),#37798,.T.);
#39928=ADVANCED_FACE('',(#4125),#571,.T.);
#39929=ADVANCED_FACE('',(#4126),#1002,.T.);
#39930=ADVANCED_FACE('',(#4127),#572,.T.);
#39931=ADVANCED_FACE('',(#4128),#37799,.F.);
#39932=ADVANCED_FACE('',(#4129),#37800,.T.);
#39933=ADVANCED_FACE('',(#4130),#1003,.T.);
#39934=ADVANCED_FACE('',(#4131),#1646,.F.);
#39935=ADVANCED_FACE('',(#4132),#37801,.T.);
#39936=ADVANCED_FACE('',(#4133),#1004,.T.);
#39937=ADVANCED_FACE('',(#4134),#1647,.F.);
#39938=ADVANCED_FACE('',(#4135),#1005,.T.);
#39939=ADVANCED_FACE('',(#4136),#37802,.T.);
#39940=ADVANCED_FACE('',(#4137),#37803,.T.);
#39941=ADVANCED_FACE('',(#4138),#1006,.T.);
#39942=ADVANCED_FACE('',(#4139),#1648,.F.);
#39943=ADVANCED_FACE('',(#4140),#1649,.F.);
#39944=ADVANCED_FACE('',(#4141),#37804,.T.);
#39945=ADVANCED_FACE('',(#4142),#37805,.T.);
#39946=ADVANCED_FACE('',(#4143),#1007,.T.);
#39947=ADVANCED_FACE('',(#4144),#37806,.T.);
#39948=ADVANCED_FACE('',(#4145),#37807,.T.);
#39949=ADVANCED_FACE('',(#4146),#1008,.T.);
#39950=ADVANCED_FACE('',(#4147),#1650,.F.);
#39951=ADVANCED_FACE('',(#4148),#1651,.F.);
#39952=ADVANCED_FACE('',(#4149,#1081),#37808,.T.);
#39953=ADVANCED_FACE('',(#4150),#37809,.T.);
#39954=ADVANCED_FACE('',(#4151),#1652,.T.);
#39955=ADVANCED_FACE('',(#4152),#1653,.F.);
#39956=ADVANCED_FACE('',(#4153),#1654,.T.);
#39957=ADVANCED_FACE('',(#4154),#748,.T.);
#39958=ADVANCED_FACE('',(#4155),#37810,.T.);
#39959=ADVANCED_FACE('',(#4156),#1655,.T.);
#39960=ADVANCED_FACE('',(#4157,#1082),#37811,.T.);
#39961=ADVANCED_FACE('',(#4158),#37812,.T.);
#39962=ADVANCED_FACE('',(#4159),#1656,.T.);
#39963=ADVANCED_FACE('',(#4160),#749,.T.);
#39964=ADVANCED_FACE('',(#4161),#1657,.T.);
#39965=ADVANCED_FACE('',(#4162,#1083),#37813,.T.);
#39966=ADVANCED_FACE('',(#4163),#37814,.T.);
#39967=ADVANCED_FACE('',(#4164),#1658,.T.);
#39968=ADVANCED_FACE('',(#4165),#750,.T.);
#39969=ADVANCED_FACE('',(#4166),#1659,.T.);
#39970=ADVANCED_FACE('',(#4167,#1084),#37815,.T.);
#39971=ADVANCED_FACE('',(#4168),#37816,.T.);
#39972=ADVANCED_FACE('',(#4169),#1660,.T.);
#39973=ADVANCED_FACE('',(#4170),#751,.T.);
#39974=ADVANCED_FACE('',(#4171),#1661,.T.);
#39975=ADVANCED_FACE('',(#4172,#1085),#37817,.T.);
#39976=ADVANCED_FACE('',(#4173),#37818,.T.);
#39977=ADVANCED_FACE('',(#4174),#1662,.T.);
#39978=ADVANCED_FACE('',(#4175),#752,.T.);
#39979=ADVANCED_FACE('',(#4176),#1663,.T.);
#39980=ADVANCED_FACE('',(#4177,#1086),#37819,.T.);
#39981=ADVANCED_FACE('',(#4178),#37820,.T.);
#39982=ADVANCED_FACE('',(#4179),#1664,.T.);
#39983=ADVANCED_FACE('',(#4180),#753,.T.);
#39984=ADVANCED_FACE('',(#4181),#1665,.T.);
#39985=ADVANCED_FACE('',(#4182,#1087),#37821,.T.);
#39986=ADVANCED_FACE('',(#4183),#37822,.T.);
#39987=ADVANCED_FACE('',(#4184),#1666,.T.);
#39988=ADVANCED_FACE('',(#4185),#754,.T.);
#39989=ADVANCED_FACE('',(#4186),#1667,.T.);
#39990=ADVANCED_FACE('',(#4187,#1088),#37823,.T.);
#39991=ADVANCED_FACE('',(#4188),#37824,.T.);
#39992=ADVANCED_FACE('',(#4189),#1668,.T.);
#39993=ADVANCED_FACE('',(#4190),#755,.T.);
#39994=ADVANCED_FACE('',(#4191),#1669,.T.);
#39995=ADVANCED_FACE('',(#4192,#1089),#37825,.T.);
#39996=ADVANCED_FACE('',(#4193),#37826,.T.);
#39997=ADVANCED_FACE('',(#4194),#1670,.T.);
#39998=ADVANCED_FACE('',(#4195),#756,.T.);
#39999=ADVANCED_FACE('',(#4196),#1671,.T.);
#40000=ADVANCED_FACE('',(#4197,#1090),#37827,.T.);
#40001=ADVANCED_FACE('',(#4198),#37828,.T.);
#40002=ADVANCED_FACE('',(#4199),#1672,.T.);
#40003=ADVANCED_FACE('',(#4200),#757,.T.);
#40004=ADVANCED_FACE('',(#4201),#1673,.T.);
#40005=ADVANCED_FACE('',(#4202,#1091),#37829,.T.);
#40006=ADVANCED_FACE('',(#4203),#37830,.T.);
#40007=ADVANCED_FACE('',(#4204),#1674,.T.);
#40008=ADVANCED_FACE('',(#4205),#758,.T.);
#40009=ADVANCED_FACE('',(#4206),#1675,.T.);
#40010=ADVANCED_FACE('',(#4207,#1092),#37831,.T.);
#40011=ADVANCED_FACE('',(#4208),#37832,.T.);
#40012=ADVANCED_FACE('',(#4209),#1676,.T.);
#40013=ADVANCED_FACE('',(#4210),#759,.T.);
#40014=ADVANCED_FACE('',(#4211),#1677,.T.);
#40015=ADVANCED_FACE('',(#4212,#1093),#37833,.T.);
#40016=ADVANCED_FACE('',(#4213),#37834,.T.);
#40017=ADVANCED_FACE('',(#4214),#1678,.T.);
#40018=ADVANCED_FACE('',(#4215),#760,.T.);
#40019=ADVANCED_FACE('',(#4216),#1679,.T.);
#40020=ADVANCED_FACE('',(#4217,#1094),#37835,.T.);
#40021=ADVANCED_FACE('',(#4218),#37836,.T.);
#40022=ADVANCED_FACE('',(#4219),#1680,.T.);
#40023=ADVANCED_FACE('',(#4220),#761,.T.);
#40024=ADVANCED_FACE('',(#4221),#1681,.T.);
#40025=ADVANCED_FACE('',(#4222,#1095),#37837,.T.);
#40026=ADVANCED_FACE('',(#4223),#37838,.T.);
#40027=ADVANCED_FACE('',(#4224),#1682,.T.);
#40028=ADVANCED_FACE('',(#4225),#762,.T.);
#40029=ADVANCED_FACE('',(#4226),#1683,.T.);
#40030=ADVANCED_FACE('',(#4227,#1096),#37839,.T.);
#40031=ADVANCED_FACE('',(#4228),#37840,.T.);
#40032=ADVANCED_FACE('',(#4229),#1684,.T.);
#40033=ADVANCED_FACE('',(#4230),#763,.T.);
#40034=ADVANCED_FACE('',(#4231),#1685,.T.);
#40035=ADVANCED_FACE('',(#4232,#1097),#37841,.T.);
#40036=ADVANCED_FACE('',(#4233),#37842,.T.);
#40037=ADVANCED_FACE('',(#4234),#1686,.T.);
#40038=ADVANCED_FACE('',(#4235),#764,.T.);
#40039=ADVANCED_FACE('',(#4236),#1687,.T.);
#40040=ADVANCED_FACE('',(#4237,#1098),#37843,.T.);
#40041=ADVANCED_FACE('',(#4238),#37844,.T.);
#40042=ADVANCED_FACE('',(#4239),#1688,.T.);
#40043=ADVANCED_FACE('',(#4240),#765,.T.);
#40044=ADVANCED_FACE('',(#4241),#1689,.T.);
#40045=ADVANCED_FACE('',(#4242,#1099),#37845,.T.);
#40046=ADVANCED_FACE('',(#4243),#37846,.T.);
#40047=ADVANCED_FACE('',(#4244),#1690,.T.);
#40048=ADVANCED_FACE('',(#4245),#766,.T.);
#40049=ADVANCED_FACE('',(#4246),#1691,.T.);
#40050=ADVANCED_FACE('',(#4247,#1100),#37847,.T.);
#40051=ADVANCED_FACE('',(#4248),#37848,.T.);
#40052=ADVANCED_FACE('',(#4249),#1692,.T.);
#40053=ADVANCED_FACE('',(#4250),#767,.T.);
#40054=ADVANCED_FACE('',(#4251),#1693,.T.);
#40055=ADVANCED_FACE('',(#4252,#1101),#37849,.T.);
#40056=ADVANCED_FACE('',(#4253),#37850,.T.);
#40057=ADVANCED_FACE('',(#4254),#1694,.T.);
#40058=ADVANCED_FACE('',(#4255),#768,.T.);
#40059=ADVANCED_FACE('',(#4256),#1695,.T.);
#40060=ADVANCED_FACE('',(#4257,#1102),#37851,.T.);
#40061=ADVANCED_FACE('',(#4258),#37852,.T.);
#40062=ADVANCED_FACE('',(#4259),#1696,.T.);
#40063=ADVANCED_FACE('',(#4260),#769,.T.);
#40064=ADVANCED_FACE('',(#4261),#1697,.T.);
#40065=ADVANCED_FACE('',(#4262,#1103),#37853,.T.);
#40066=ADVANCED_FACE('',(#4263),#37854,.T.);
#40067=ADVANCED_FACE('',(#4264),#1698,.T.);
#40068=ADVANCED_FACE('',(#4265),#770,.T.);
#40069=ADVANCED_FACE('',(#4266),#1699,.T.);
#40070=ADVANCED_FACE('',(#4267,#1104),#37855,.T.);
#40071=ADVANCED_FACE('',(#4268),#37856,.T.);
#40072=ADVANCED_FACE('',(#4269),#1700,.T.);
#40073=ADVANCED_FACE('',(#4270),#771,.T.);
#40074=ADVANCED_FACE('',(#4271),#1701,.T.);
#40075=ADVANCED_FACE('',(#4272,#1105),#37857,.T.);
#40076=ADVANCED_FACE('',(#4273),#772,.T.);
#40077=ADVANCED_FACE('',(#4274),#37858,.T.);
#40078=ADVANCED_FACE('',(#4275),#1702,.T.);
#40079=ADVANCED_FACE('',(#4276,#1106),#37859,.T.);
#40080=ADVANCED_FACE('',(#4277),#37860,.T.);
#40081=ADVANCED_FACE('',(#4278),#1703,.T.);
#40082=ADVANCED_FACE('',(#4279),#1009,.T.);
#40083=ADVANCED_FACE('',(#4280,#1107),#1704,.T.);
#40084=ADVANCED_FACE('',(#4281),#37861,.T.);
#40085=ADVANCED_FACE('',(#4282),#773,.T.);
#40086=ADVANCED_FACE('',(#4283),#1705,.F.);
#40087=ADVANCED_FACE('',(#4284),#1706,.T.);
#40088=ADVANCED_FACE('',(#4285),#1707,.F.);
#40089=ADVANCED_FACE('',(#4286),#1708,.F.);
#40090=ADVANCED_FACE('',(#4287),#1709,.F.);
#40091=ADVANCED_FACE('',(#4288),#1710,.F.);
#40092=ADVANCED_FACE('',(#4289),#1711,.F.);
#40093=ADVANCED_FACE('',(#4290),#1712,.F.);
#40094=ADVANCED_FACE('',(#4291),#1713,.F.);
#40095=ADVANCED_FACE('',(#4292),#1714,.F.);
#40096=ADVANCED_FACE('',(#4293),#1715,.F.);
#40097=ADVANCED_FACE('',(#4294),#1716,.F.);
#40098=ADVANCED_FACE('',(#4295),#1717,.F.);
#40099=ADVANCED_FACE('',(#4296),#1718,.F.);
#40100=ADVANCED_FACE('',(#4297),#1719,.F.);
#40101=ADVANCED_FACE('',(#4298),#1720,.F.);
#40102=ADVANCED_FACE('',(#4299),#1721,.F.);
#40103=ADVANCED_FACE('',(#4300),#1722,.F.);
#40104=ADVANCED_FACE('',(#4301),#1723,.F.);
#40105=ADVANCED_FACE('',(#4302),#1724,.F.);
#40106=ADVANCED_FACE('',(#4303),#1725,.F.);
#40107=ADVANCED_FACE('',(#4304),#1726,.F.);
#40108=ADVANCED_FACE('',(#4305),#1727,.F.);
#40109=ADVANCED_FACE('',(#4306),#1728,.F.);
#40110=ADVANCED_FACE('',(#4307),#1729,.F.);
#40111=ADVANCED_FACE('',(#4308),#1730,.F.);
#40112=ADVANCED_FACE('',(#4309),#37862,.T.);
#40113=ADVANCED_FACE('',(#4310),#1731,.F.);
#40114=ADVANCED_FACE('',(#4311),#1732,.F.);
#40115=ADVANCED_FACE('',(#4312),#1733,.F.);
#40116=ADVANCED_FACE('',(#4313),#1734,.F.);
#40117=ADVANCED_FACE('',(#4314),#37863,.F.);
#40118=ADVANCED_FACE('',(#4315),#774,.T.);
#40119=ADVANCED_FACE('',(#4316),#1735,.T.);
#40357=CLOSED_SHELL('',(#39891,#39892,#39893,#39894,#39895,#39896,#39897,
#39898,#39899,#39900,#39901,#39902,#39903,#39904,#39905,#39906,#39907,#39908,
#39909,#39910,#39911,#39912,#39913,#39914,#39915,#39916,#39917,#39918,#39919,
#39920,#39921,#39922,#39923,#39924,#39925,#39926,#39927,#39928,#39929,#39930,
#39931,#39932,#39933,#39934,#39935,#39936,#39937,#39938,#39939,#39940,#39941,
#39942,#39943,#39944,#39945,#39946,#39947,#39948,#39949,#39950,#39951,#39952,
#39953,#39954,#39955,#39956,#39957,#39958,#39959,#39960,#39961,#39962,#39963,
#39964,#39965,#39966,#39967,#39968,#39969,#39970,#39971,#39972,#39973,#39974,
#39975,#39976,#39977,#39978,#39979,#39980,#39981,#39982,#39983,#39984,#39985,
#39986,#39987,#39988,#39989,#39990,#39991,#39992,#39993,#39994,#39995,#39996,
#39997,#39998,#39999,#40000,#40001,#40002,#40003,#40004,#40005,#40006,#40007,
#40008,#40009,#40010,#40011,#40012,#40013,#40014,#40015,#40016,#40017,#40018,
#40019,#40020,#40021,#40022,#40023,#40024,#40025,#40026,#40027,#40028,#40029,
#40030,#40031,#40032,#40033,#40034,#40035,#40036,#40037,#40038,#40039,#40040,
#40041,#40042,#40043,#40044,#40045,#40046,#40047,#40048,#40049,#40050,#40051,
#40052,#40053,#40054,#40055,#40056,#40057,#40058,#40059,#40060,#40061,#40062,
#40063,#40064,#40065,#40066,#40067,#40068,#40069,#40070,#40071,#40072,#40073,
#40074,#40075,#40076,#40077,#40078,#40079,#40080,#40081,#40082,#40083,#40084,
#40085,#40086,#40087,#40088,#40089,#40090,#40091,#40092,#40093,#40094,#40095,
#40096,#40097,#40098,#40099,#40100,#40101,#40102,#40103,#40104,#40105,#40106,
#40107,#40108,#40109,#40110,#40111,#40112,#40113,#40114,#40115,#40116,#40117,
#40118,#40119));
#44271=AXIS2_PLACEMENT_3D('',#86928,#54726,#54727);
#44272=AXIS2_PLACEMENT_3D('',#86929,#54728,#54729);
#44273=AXIS2_PLACEMENT_3D('',#86931,#54730,#54731);
#44274=AXIS2_PLACEMENT_3D('',#86933,#54732,#54733);
#44275=AXIS2_PLACEMENT_3D('',#86935,#54734,#54735);
#44276=AXIS2_PLACEMENT_3D('',#86936,#54736,#54737);
#44277=AXIS2_PLACEMENT_3D('',#86937,#54738,#54739);
#44278=AXIS2_PLACEMENT_3D('',#86940,#54741,#54742);
#44279=AXIS2_PLACEMENT_3D('',#86941,#54743,#54744);
#44280=AXIS2_PLACEMENT_3D('',#86943,#54745,#54746);
#44281=AXIS2_PLACEMENT_3D('',#86944,#54747,#54748);
#44282=AXIS2_PLACEMENT_3D('',#86946,#54749,#54750);
#44283=AXIS2_PLACEMENT_3D('',#86948,#54751,#54752);
#44284=AXIS2_PLACEMENT_3D('',#86950,#54753,#54754);
#44285=AXIS2_PLACEMENT_3D('',#86951,#54755,#54756);
#44286=AXIS2_PLACEMENT_3D('',#86952,#54757,#54758);
#44287=AXIS2_PLACEMENT_3D('',#86955,#54760,#54761);
#44288=AXIS2_PLACEMENT_3D('',#86956,#54762,#54763);
#44289=AXIS2_PLACEMENT_3D('',#86957,#54764,#54765);
#44290=AXIS2_PLACEMENT_3D('',#86959,#54766,#54767);
#44291=AXIS2_PLACEMENT_3D('',#86961,#54768,#54769);
#44292=AXIS2_PLACEMENT_3D('',#86963,#54770,#54771);
#44293=AXIS2_PLACEMENT_3D('',#86964,#54772,#54773);
#44294=AXIS2_PLACEMENT_3D('',#86965,#54774,#54775);
#44295=AXIS2_PLACEMENT_3D('',#86968,#54777,#54778);
#44296=AXIS2_PLACEMENT_3D('',#86969,#54779,#54780);
#44297=AXIS2_PLACEMENT_3D('',#86970,#54781,#54782);
#44298=AXIS2_PLACEMENT_3D('',#86973,#54783,#54784);
#44299=AXIS2_PLACEMENT_3D('',#86974,#54785,#54786);
#44300=AXIS2_PLACEMENT_3D('',#86976,#54787,#54788);
#44301=AXIS2_PLACEMENT_3D('',#86978,#54789,#54790);
#44302=AXIS2_PLACEMENT_3D('',#86979,#54791,#54792);
#44303=AXIS2_PLACEMENT_3D('',#86980,#54793,#54794);
#44304=AXIS2_PLACEMENT_3D('',#86984,#54796,#54797);
#44305=AXIS2_PLACEMENT_3D('',#86985,#54798,#54799);
#44306=AXIS2_PLACEMENT_3D('',#86986,#54800,#54801);
#44307=AXIS2_PLACEMENT_3D('',#86989,#54802,#54803);
#44308=AXIS2_PLACEMENT_3D('',#86991,#54804,#54805);
#44309=AXIS2_PLACEMENT_3D('',#86993,#54806,#54807);
#44310=AXIS2_PLACEMENT_3D('',#86995,#54808,#54809);
#44311=AXIS2_PLACEMENT_3D('',#86997,#54810,#54811);
#44312=AXIS2_PLACEMENT_3D('',#86999,#54812,#54813);
#44313=AXIS2_PLACEMENT_3D('',#87001,#54815,#54816);
#44314=AXIS2_PLACEMENT_3D('',#87002,#54817,#54818);
#44315=AXIS2_PLACEMENT_3D('',#87004,#54819,#54820);
#44316=AXIS2_PLACEMENT_3D('',#87006,#54821,#54822);
#44317=AXIS2_PLACEMENT_3D('',#87007,#54823,#54824);
#44318=AXIS2_PLACEMENT_3D('',#87008,#54825,#54826);
#44319=AXIS2_PLACEMENT_3D('',#87012,#54828,#54829);
#44320=AXIS2_PLACEMENT_3D('',#87013,#54830,#54831);
#44321=AXIS2_PLACEMENT_3D('',#87014,#54832,#54833);
#44322=AXIS2_PLACEMENT_3D('',#87017,#54834,#54835);
#44323=AXIS2_PLACEMENT_3D('',#87021,#54837,#54838);
#44324=AXIS2_PLACEMENT_3D('',#87023,#54840,#54841);
#44325=AXIS2_PLACEMENT_3D('',#87025,#54842,#54843);
#44326=AXIS2_PLACEMENT_3D('',#87027,#54844,#54845);
#44327=AXIS2_PLACEMENT_3D('',#87029,#54846,#54847);
#44328=AXIS2_PLACEMENT_3D('',#87030,#54848,#54849);
#44329=AXIS2_PLACEMENT_3D('',#87031,#54850,#54851);
#44330=AXIS2_PLACEMENT_3D('',#87032,#54852,#54853);
#44331=AXIS2_PLACEMENT_3D('',#87033,#54854,#54855);
#44332=AXIS2_PLACEMENT_3D('',#87035,#54856,#54857);
#44333=AXIS2_PLACEMENT_3D('',#87039,#54859,#54860);
#44334=AXIS2_PLACEMENT_3D('',#87041,#54862,#54863);
#44335=AXIS2_PLACEMENT_3D('',#87042,#54864,#54865);
#44336=AXIS2_PLACEMENT_3D('',#87043,#54866,#54867);
#44337=AXIS2_PLACEMENT_3D('',#87045,#54868,#54869);
#44338=AXIS2_PLACEMENT_3D('',#87048,#54871,#54872);
#44339=AXIS2_PLACEMENT_3D('',#87049,#54873,#54874);
#44340=AXIS2_PLACEMENT_3D('',#87051,#54875,#54876);
#44341=AXIS2_PLACEMENT_3D('',#87052,#54877,#54878);
#44342=AXIS2_PLACEMENT_3D('',#87053,#54879,#54880);
#44343=AXIS2_PLACEMENT_3D('',#87055,#54881,#54882);
#44344=AXIS2_PLACEMENT_3D('',#87057,#54883,#54884);
#44345=AXIS2_PLACEMENT_3D('',#87059,#54885,#54886);
#44346=AXIS2_PLACEMENT_3D('',#87061,#54887,#54888);
#44347=AXIS2_PLACEMENT_3D('',#87062,#54889,#54890);
#44348=AXIS2_PLACEMENT_3D('',#87063,#54891,#54892);
#44349=AXIS2_PLACEMENT_3D('',#87065,#54893,#54894);
#44350=AXIS2_PLACEMENT_3D('',#87066,#54895,#54896);
#44351=AXIS2_PLACEMENT_3D('',#87067,#54897,#54898);
#44352=AXIS2_PLACEMENT_3D('',#87069,#54899,#54900);
#44353=AXIS2_PLACEMENT_3D('',#87071,#54902,#54903);
#44354=AXIS2_PLACEMENT_3D('',#87073,#54904,#54905);
#44355=AXIS2_PLACEMENT_3D('',#87076,#54907,#54908);
#44356=AXIS2_PLACEMENT_3D('',#87077,#54909,#54910);
#44357=AXIS2_PLACEMENT_3D('',#87078,#54911,#54912);
#44358=AXIS2_PLACEMENT_3D('',#87079,#54913,#54914);
#44359=AXIS2_PLACEMENT_3D('',#87081,#54915,#54916);
#44360=AXIS2_PLACEMENT_3D('',#87084,#54918,#54919);
#44361=AXIS2_PLACEMENT_3D('',#87085,#54920,#54921);
#44362=AXIS2_PLACEMENT_3D('',#87086,#54922,#54923);
#44363=AXIS2_PLACEMENT_3D('',#87087,#54924,#54925);
#44364=AXIS2_PLACEMENT_3D('',#87088,#54926,#54927);
#44365=AXIS2_PLACEMENT_3D('',#87089,#54928,#54929);
#44366=AXIS2_PLACEMENT_3D('',#87111,#54932,#54933);
#44367=AXIS2_PLACEMENT_3D('',#87153,#54937,#54938);
#44368=AXIS2_PLACEMENT_3D('',#87172,#54940,#54941);
#44369=AXIS2_PLACEMENT_3D('',#87174,#54942,#54943);
#44370=AXIS2_PLACEMENT_3D('',#87176,#54944,#54945);
#44371=AXIS2_PLACEMENT_3D('',#87178,#54947,#54948);
#44372=AXIS2_PLACEMENT_3D('',#87179,#54949,#54950);
#44373=AXIS2_PLACEMENT_3D('',#87180,#54951,#54952);
#44374=AXIS2_PLACEMENT_3D('',#87182,#54953,#54954);
#44375=AXIS2_PLACEMENT_3D('',#87183,#54955,#54956);
#44376=AXIS2_PLACEMENT_3D('',#87184,#54957,#54958);
#44377=AXIS2_PLACEMENT_3D('',#87186,#54959,#54960);
#44378=AXIS2_PLACEMENT_3D('',#87188,#54962,#54963);
#44379=AXIS2_PLACEMENT_3D('',#87190,#54964,#54965);
#44380=AXIS2_PLACEMENT_3D('',#87193,#54967,#54968);
#44381=AXIS2_PLACEMENT_3D('',#87194,#54969,#54970);
#44382=AXIS2_PLACEMENT_3D('',#87195,#54971,#54972);
#44383=AXIS2_PLACEMENT_3D('',#87196,#54973,#54974);
#44384=AXIS2_PLACEMENT_3D('',#87198,#54975,#54976);
#44385=AXIS2_PLACEMENT_3D('',#87199,#54977,#54978);
#44386=AXIS2_PLACEMENT_3D('',#87200,#54979,#54980);
#44387=AXIS2_PLACEMENT_3D('',#87201,#54981,#54982);
#44388=AXIS2_PLACEMENT_3D('',#87202,#54983,#54984);
#44389=AXIS2_PLACEMENT_3D('',#87205,#54986,#54987);
#44390=AXIS2_PLACEMENT_3D('',#87206,#54988,#54989);
#44391=AXIS2_PLACEMENT_3D('',#87207,#54990,#54991);
#44392=AXIS2_PLACEMENT_3D('',#87208,#54992,#54993);
#44393=AXIS2_PLACEMENT_3D('',#87209,#54994,#54995);
#44394=AXIS2_PLACEMENT_3D('',#87211,#54996,#54997);
#44395=AXIS2_PLACEMENT_3D('',#87212,#54998,#54999);
#44396=AXIS2_PLACEMENT_3D('',#87213,#55000,#55001);
#44397=AXIS2_PLACEMENT_3D('',#87214,#55002,#55003);
#44398=AXIS2_PLACEMENT_3D('',#87216,#55004,#55005);
#44399=AXIS2_PLACEMENT_3D('',#87218,#55007,#55008);
#44400=AXIS2_PLACEMENT_3D('',#87219,#55009,#55010);
#44401=AXIS2_PLACEMENT_3D('',#87220,#55011,#55012);
#44402=AXIS2_PLACEMENT_3D('',#87221,#55013,#55014);
#44403=AXIS2_PLACEMENT_3D('',#87241,#55015,#55016);
#44404=AXIS2_PLACEMENT_3D('',#87257,#55017,#55018);
#44405=AXIS2_PLACEMENT_3D('',#87270,#55021,#55022);
#44406=AXIS2_PLACEMENT_3D('',#87281,#55025,#55026);
#44407=AXIS2_PLACEMENT_3D('',#87282,#55027,#55028);
#44408=AXIS2_PLACEMENT_3D('',#87293,#55029,#55030);
#44409=AXIS2_PLACEMENT_3D('',#87302,#55031,#55032);
#44410=AXIS2_PLACEMENT_3D('',#87305,#55035,#55036);
#44411=AXIS2_PLACEMENT_3D('',#87306,#55037,#55038);
#44412=AXIS2_PLACEMENT_3D('',#87307,#55039,#55040);
#44413=AXIS2_PLACEMENT_3D('',#87308,#55041,#55042);
#44414=AXIS2_PLACEMENT_3D('',#87311,#55044,#55045);
#44415=AXIS2_PLACEMENT_3D('',#87312,#55046,#55047);
#44416=AXIS2_PLACEMENT_3D('',#87332,#55048,#55049);
#44417=AXIS2_PLACEMENT_3D('',#87348,#55050,#55051);
#44418=AXIS2_PLACEMENT_3D('',#87359,#55053,#55054);
#44419=AXIS2_PLACEMENT_3D('',#87368,#55056,#55057);
#44420=AXIS2_PLACEMENT_3D('',#87369,#55058,#55059);
#44421=AXIS2_PLACEMENT_3D('',#87380,#55060,#55061);
#44422=AXIS2_PLACEMENT_3D('',#87389,#55062,#55063);
#44423=AXIS2_PLACEMENT_3D('',#87392,#55066,#55067);
#44424=AXIS2_PLACEMENT_3D('',#87393,#55068,#55069);
#44425=AXIS2_PLACEMENT_3D('',#87396,#55070,#55071);
#44426=AXIS2_PLACEMENT_3D('',#87400,#55073,#55074);
#44427=AXIS2_PLACEMENT_3D('',#87404,#55076,#55077);
#44428=AXIS2_PLACEMENT_3D('',#87413,#55078,#55079);
#44429=AXIS2_PLACEMENT_3D('',#87417,#55081,#55082);
#44430=AXIS2_PLACEMENT_3D('',#87419,#55084,#55085);
#44431=AXIS2_PLACEMENT_3D('',#87420,#55086,#55087);
#44432=AXIS2_PLACEMENT_3D('',#87421,#55088,#55089);
#44433=AXIS2_PLACEMENT_3D('',#87422,#55090,#55091);
#44434=AXIS2_PLACEMENT_3D('',#87423,#55092,#55093);
#44435=AXIS2_PLACEMENT_3D('',#87433,#55096,#55097);
#44436=AXIS2_PLACEMENT_3D('',#87434,#55098,#55099);
#44437=AXIS2_PLACEMENT_3D('',#87438,#55101,#55102);
#44438=AXIS2_PLACEMENT_3D('',#87440,#55103,#55104);
#44439=AXIS2_PLACEMENT_3D('',#87442,#55105,#55106);
#44440=AXIS2_PLACEMENT_3D('',#87446,#55108,#55109);
#44441=AXIS2_PLACEMENT_3D('',#87448,#55110,#55111);
#44442=AXIS2_PLACEMENT_3D('',#87450,#55112,#55113);
#44443=AXIS2_PLACEMENT_3D('',#87454,#55115,#55116);
#44444=AXIS2_PLACEMENT_3D('',#87456,#55117,#55118);
#44445=AXIS2_PLACEMENT_3D('',#87458,#55119,#55120);
#44446=AXIS2_PLACEMENT_3D('',#87462,#55122,#55123);
#44447=AXIS2_PLACEMENT_3D('',#87464,#55124,#55125);
#44448=AXIS2_PLACEMENT_3D('',#87466,#55126,#55127);
#44449=AXIS2_PLACEMENT_3D('',#87470,#55129,#55130);
#44450=AXIS2_PLACEMENT_3D('',#87472,#55131,#55132);
#44451=AXIS2_PLACEMENT_3D('',#87474,#55133,#55134);
#44452=AXIS2_PLACEMENT_3D('',#87478,#55136,#55137);
#44453=AXIS2_PLACEMENT_3D('',#87480,#55138,#55139);
#44454=AXIS2_PLACEMENT_3D('',#87482,#55140,#55141);
#44455=AXIS2_PLACEMENT_3D('',#87486,#55143,#55144);
#44456=AXIS2_PLACEMENT_3D('',#87488,#55145,#55146);
#44457=AXIS2_PLACEMENT_3D('',#87490,#55147,#55148);
#44458=AXIS2_PLACEMENT_3D('',#87494,#55150,#55151);
#44459=AXIS2_PLACEMENT_3D('',#87496,#55152,#55153);
#44460=AXIS2_PLACEMENT_3D('',#87498,#55154,#55155);
#44461=AXIS2_PLACEMENT_3D('',#87502,#55157,#55158);
#44462=AXIS2_PLACEMENT_3D('',#87504,#55159,#55160);
#44463=AXIS2_PLACEMENT_3D('',#87506,#55161,#55162);
#44464=AXIS2_PLACEMENT_3D('',#87510,#55164,#55165);
#44465=AXIS2_PLACEMENT_3D('',#87512,#55166,#55167);
#44466=AXIS2_PLACEMENT_3D('',#87514,#55168,#55169);
#44467=AXIS2_PLACEMENT_3D('',#87518,#55171,#55172);
#44468=AXIS2_PLACEMENT_3D('',#87520,#55173,#55174);
#44469=AXIS2_PLACEMENT_3D('',#87522,#55175,#55176);
#44470=AXIS2_PLACEMENT_3D('',#87526,#55178,#55179);
#44471=AXIS2_PLACEMENT_3D('',#87528,#55180,#55181);
#44472=AXIS2_PLACEMENT_3D('',#87530,#55182,#55183);
#44473=AXIS2_PLACEMENT_3D('',#87534,#55185,#55186);
#44474=AXIS2_PLACEMENT_3D('',#87536,#55187,#55188);
#44475=AXIS2_PLACEMENT_3D('',#87538,#55189,#55190);
#44476=AXIS2_PLACEMENT_3D('',#87542,#55192,#55193);
#44477=AXIS2_PLACEMENT_3D('',#87544,#55194,#55195);
#44478=AXIS2_PLACEMENT_3D('',#87546,#55196,#55197);
#44479=AXIS2_PLACEMENT_3D('',#87550,#55199,#55200);
#44480=AXIS2_PLACEMENT_3D('',#87552,#55201,#55202);
#44481=AXIS2_PLACEMENT_3D('',#87554,#55203,#55204);
#44482=AXIS2_PLACEMENT_3D('',#87558,#55206,#55207);
#44483=AXIS2_PLACEMENT_3D('',#87560,#55208,#55209);
#44484=AXIS2_PLACEMENT_3D('',#87562,#55210,#55211);
#44485=AXIS2_PLACEMENT_3D('',#87566,#55213,#55214);
#44486=AXIS2_PLACEMENT_3D('',#87568,#55215,#55216);
#44487=AXIS2_PLACEMENT_3D('',#87570,#55217,#55218);
#44488=AXIS2_PLACEMENT_3D('',#87574,#55220,#55221);
#44489=AXIS2_PLACEMENT_3D('',#87576,#55222,#55223);
#44490=AXIS2_PLACEMENT_3D('',#87578,#55224,#55225);
#44491=AXIS2_PLACEMENT_3D('',#87582,#55227,#55228);
#44492=AXIS2_PLACEMENT_3D('',#87584,#55229,#55230);
#44493=AXIS2_PLACEMENT_3D('',#87586,#55231,#55232);
#44494=AXIS2_PLACEMENT_3D('',#87590,#55234,#55235);
#44495=AXIS2_PLACEMENT_3D('',#87592,#55236,#55237);
#44496=AXIS2_PLACEMENT_3D('',#87594,#55238,#55239);
#44497=AXIS2_PLACEMENT_3D('',#87598,#55241,#55242);
#44498=AXIS2_PLACEMENT_3D('',#87600,#55243,#55244);
#44499=AXIS2_PLACEMENT_3D('',#87602,#55245,#55246);
#44500=AXIS2_PLACEMENT_3D('',#87606,#55248,#55249);
#44501=AXIS2_PLACEMENT_3D('',#87608,#55250,#55251);
#44502=AXIS2_PLACEMENT_3D('',#87610,#55252,#55253);
#44503=AXIS2_PLACEMENT_3D('',#87614,#55255,#55256);
#44504=AXIS2_PLACEMENT_3D('',#87616,#55257,#55258);
#44505=AXIS2_PLACEMENT_3D('',#87618,#55259,#55260);
#44506=AXIS2_PLACEMENT_3D('',#87622,#55262,#55263);
#44507=AXIS2_PLACEMENT_3D('',#87624,#55264,#55265);
#44508=AXIS2_PLACEMENT_3D('',#87626,#55266,#55267);
#44509=AXIS2_PLACEMENT_3D('',#87630,#55269,#55270);
#44510=AXIS2_PLACEMENT_3D('',#87632,#55271,#55272);
#44511=AXIS2_PLACEMENT_3D('',#87634,#55273,#55274);
#44512=AXIS2_PLACEMENT_3D('',#87636,#55276,#55277);
#44513=AXIS2_PLACEMENT_3D('',#87637,#55278,#55279);
#44514=AXIS2_PLACEMENT_3D('',#87640,#55280,#55281);
#44515=AXIS2_PLACEMENT_3D('',#87649,#55283,#55284);
#44516=AXIS2_PLACEMENT_3D('',#87650,#55285,#55286);
#44517=AXIS2_PLACEMENT_3D('',#87653,#55287,#55288);
#44518=AXIS2_PLACEMENT_3D('',#87664,#55291,#55292);
#44519=AXIS2_PLACEMENT_3D('',#87668,#55294,#55295);
#44520=AXIS2_PLACEMENT_3D('',#87670,#55297,#55298);
#44521=AXIS2_PLACEMENT_3D('',#87671,#55299,#55300);
#44522=AXIS2_PLACEMENT_3D('',#87672,#55301,#55302);
#44523=AXIS2_PLACEMENT_3D('',#87673,#55303,#55304);
#44524=AXIS2_PLACEMENT_3D('',#87674,#55305,#55306);
#44525=AXIS2_PLACEMENT_3D('',#87675,#55307,#55308);
#44526=AXIS2_PLACEMENT_3D('',#87676,#55309,#55310);
#44527=AXIS2_PLACEMENT_3D('',#87679,#55311,#55312);
#44528=AXIS2_PLACEMENT_3D('',#87690,#55315,#55316);
#44529=AXIS2_PLACEMENT_3D('',#87694,#55318,#55319);
#44530=AXIS2_PLACEMENT_3D('',#87696,#55321,#55322);
#44531=AXIS2_PLACEMENT_3D('',#87697,#55323,#55324);
#44532=AXIS2_PLACEMENT_3D('',#87698,#55325,#55326);
#44533=AXIS2_PLACEMENT_3D('',#87699,#55327,#55328);
#44534=AXIS2_PLACEMENT_3D('',#87700,#55329,#55330);
#44535=AXIS2_PLACEMENT_3D('',#87701,#55331,#55332);
#44536=AXIS2_PLACEMENT_3D('',#87702,#55333,#55334);
#44537=AXIS2_PLACEMENT_3D('',#87705,#55335,#55336);
#44538=AXIS2_PLACEMENT_3D('',#87716,#55339,#55340);
#44539=AXIS2_PLACEMENT_3D('',#87720,#55342,#55343);
#44540=AXIS2_PLACEMENT_3D('',#87722,#55345,#55346);
#44541=AXIS2_PLACEMENT_3D('',#87723,#55347,#55348);
#44542=AXIS2_PLACEMENT_3D('',#87724,#55349,#55350);
#44543=AXIS2_PLACEMENT_3D('',#87725,#55351,#55352);
#44544=AXIS2_PLACEMENT_3D('',#87726,#55353,#55354);
#44545=AXIS2_PLACEMENT_3D('',#87727,#55355,#55356);
#44546=AXIS2_PLACEMENT_3D('',#87728,#55357,#55358);
#44547=AXIS2_PLACEMENT_3D('',#87731,#55359,#55360);
#44548=AXIS2_PLACEMENT_3D('',#87742,#55363,#55364);
#44549=AXIS2_PLACEMENT_3D('',#87746,#55366,#55367);
#44550=AXIS2_PLACEMENT_3D('',#87748,#55369,#55370);
#44551=AXIS2_PLACEMENT_3D('',#87749,#55371,#55372);
#44552=AXIS2_PLACEMENT_3D('',#87750,#55373,#55374);
#44553=AXIS2_PLACEMENT_3D('',#87751,#55375,#55376);
#44554=AXIS2_PLACEMENT_3D('',#87752,#55377,#55378);
#44555=AXIS2_PLACEMENT_3D('',#87753,#55379,#55380);
#44556=AXIS2_PLACEMENT_3D('',#87754,#55381,#55382);
#44557=AXIS2_PLACEMENT_3D('',#87757,#55383,#55384);
#44558=AXIS2_PLACEMENT_3D('',#87768,#55387,#55388);
#44559=AXIS2_PLACEMENT_3D('',#87772,#55390,#55391);
#44560=AXIS2_PLACEMENT_3D('',#87774,#55393,#55394);
#44561=AXIS2_PLACEMENT_3D('',#87775,#55395,#55396);
#44562=AXIS2_PLACEMENT_3D('',#87776,#55397,#55398);
#44563=AXIS2_PLACEMENT_3D('',#87777,#55399,#55400);
#44564=AXIS2_PLACEMENT_3D('',#87778,#55401,#55402);
#44565=AXIS2_PLACEMENT_3D('',#87779,#55403,#55404);
#44566=AXIS2_PLACEMENT_3D('',#87780,#55405,#55406);
#44567=AXIS2_PLACEMENT_3D('',#87783,#55407,#55408);
#44568=AXIS2_PLACEMENT_3D('',#87794,#55411,#55412);
#44569=AXIS2_PLACEMENT_3D('',#87798,#55414,#55415);
#44570=AXIS2_PLACEMENT_3D('',#87800,#55417,#55418);
#44571=AXIS2_PLACEMENT_3D('',#87801,#55419,#55420);
#44572=AXIS2_PLACEMENT_3D('',#87802,#55421,#55422);
#44573=AXIS2_PLACEMENT_3D('',#87803,#55423,#55424);
#44574=AXIS2_PLACEMENT_3D('',#87804,#55425,#55426);
#44575=AXIS2_PLACEMENT_3D('',#87805,#55427,#55428);
#44576=AXIS2_PLACEMENT_3D('',#87806,#55429,#55430);
#44577=AXIS2_PLACEMENT_3D('',#87809,#55431,#55432);
#44578=AXIS2_PLACEMENT_3D('',#87820,#55435,#55436);
#44579=AXIS2_PLACEMENT_3D('',#87824,#55438,#55439);
#44580=AXIS2_PLACEMENT_3D('',#87826,#55441,#55442);
#44581=AXIS2_PLACEMENT_3D('',#87827,#55443,#55444);
#44582=AXIS2_PLACEMENT_3D('',#87828,#55445,#55446);
#44583=AXIS2_PLACEMENT_3D('',#87829,#55447,#55448);
#44584=AXIS2_PLACEMENT_3D('',#87830,#55449,#55450);
#44585=AXIS2_PLACEMENT_3D('',#87831,#55451,#55452);
#44586=AXIS2_PLACEMENT_3D('',#87832,#55453,#55454);
#44587=AXIS2_PLACEMENT_3D('',#87835,#55455,#55456);
#44588=AXIS2_PLACEMENT_3D('',#87846,#55459,#55460);
#44589=AXIS2_PLACEMENT_3D('',#87850,#55462,#55463);
#44590=AXIS2_PLACEMENT_3D('',#87852,#55465,#55466);
#44591=AXIS2_PLACEMENT_3D('',#87853,#55467,#55468);
#44592=AXIS2_PLACEMENT_3D('',#87854,#55469,#55470);
#44593=AXIS2_PLACEMENT_3D('',#87855,#55471,#55472);
#44594=AXIS2_PLACEMENT_3D('',#87856,#55473,#55474);
#44595=AXIS2_PLACEMENT_3D('',#87857,#55475,#55476);
#44596=AXIS2_PLACEMENT_3D('',#87858,#55477,#55478);
#44597=AXIS2_PLACEMENT_3D('',#87861,#55479,#55480);
#44598=AXIS2_PLACEMENT_3D('',#87872,#55483,#55484);
#44599=AXIS2_PLACEMENT_3D('',#87876,#55486,#55487);
#44600=AXIS2_PLACEMENT_3D('',#87878,#55489,#55490);
#44601=AXIS2_PLACEMENT_3D('',#87879,#55491,#55492);
#44602=AXIS2_PLACEMENT_3D('',#87880,#55493,#55494);
#44603=AXIS2_PLACEMENT_3D('',#87881,#55495,#55496);
#44604=AXIS2_PLACEMENT_3D('',#87882,#55497,#55498);
#44605=AXIS2_PLACEMENT_3D('',#87883,#55499,#55500);
#44606=AXIS2_PLACEMENT_3D('',#87884,#55501,#55502);
#44607=AXIS2_PLACEMENT_3D('',#87887,#55503,#55504);
#44608=AXIS2_PLACEMENT_3D('',#87898,#55507,#55508);
#44609=AXIS2_PLACEMENT_3D('',#87902,#55510,#55511);
#44610=AXIS2_PLACEMENT_3D('',#87904,#55513,#55514);
#44611=AXIS2_PLACEMENT_3D('',#87905,#55515,#55516);
#44612=AXIS2_PLACEMENT_3D('',#87906,#55517,#55518);
#44613=AXIS2_PLACEMENT_3D('',#87907,#55519,#55520);
#44614=AXIS2_PLACEMENT_3D('',#87908,#55521,#55522);
#44615=AXIS2_PLACEMENT_3D('',#87909,#55523,#55524);
#44616=AXIS2_PLACEMENT_3D('',#87910,#55525,#55526);
#44617=AXIS2_PLACEMENT_3D('',#87913,#55527,#55528);
#44618=AXIS2_PLACEMENT_3D('',#87924,#55531,#55532);
#44619=AXIS2_PLACEMENT_3D('',#87928,#55534,#55535);
#44620=AXIS2_PLACEMENT_3D('',#87930,#55537,#55538);
#44621=AXIS2_PLACEMENT_3D('',#87931,#55539,#55540);
#44622=AXIS2_PLACEMENT_3D('',#87932,#55541,#55542);
#44623=AXIS2_PLACEMENT_3D('',#87933,#55543,#55544);
#44624=AXIS2_PLACEMENT_3D('',#87934,#55545,#55546);
#44625=AXIS2_PLACEMENT_3D('',#87935,#55547,#55548);
#44626=AXIS2_PLACEMENT_3D('',#87936,#55549,#55550);
#44627=AXIS2_PLACEMENT_3D('',#87939,#55551,#55552);
#44628=AXIS2_PLACEMENT_3D('',#87950,#55555,#55556);
#44629=AXIS2_PLACEMENT_3D('',#87954,#55558,#55559);
#44630=AXIS2_PLACEMENT_3D('',#87956,#55561,#55562);
#44631=AXIS2_PLACEMENT_3D('',#87957,#55563,#55564);
#44632=AXIS2_PLACEMENT_3D('',#87958,#55565,#55566);
#44633=AXIS2_PLACEMENT_3D('',#87959,#55567,#55568);
#44634=AXIS2_PLACEMENT_3D('',#87960,#55569,#55570);
#44635=AXIS2_PLACEMENT_3D('',#87961,#55571,#55572);
#44636=AXIS2_PLACEMENT_3D('',#87962,#55573,#55574);
#44637=AXIS2_PLACEMENT_3D('',#87965,#55575,#55576);
#44638=AXIS2_PLACEMENT_3D('',#87976,#55579,#55580);
#44639=AXIS2_PLACEMENT_3D('',#87980,#55582,#55583);
#44640=AXIS2_PLACEMENT_3D('',#87982,#55585,#55586);
#44641=AXIS2_PLACEMENT_3D('',#87983,#55587,#55588);
#44642=AXIS2_PLACEMENT_3D('',#87984,#55589,#55590);
#44643=AXIS2_PLACEMENT_3D('',#87985,#55591,#55592);
#44644=AXIS2_PLACEMENT_3D('',#87986,#55593,#55594);
#44645=AXIS2_PLACEMENT_3D('',#87987,#55595,#55596);
#44646=AXIS2_PLACEMENT_3D('',#87988,#55597,#55598);
#44647=AXIS2_PLACEMENT_3D('',#87991,#55599,#55600);
#44648=AXIS2_PLACEMENT_3D('',#88002,#55603,#55604);
#44649=AXIS2_PLACEMENT_3D('',#88006,#55606,#55607);
#44650=AXIS2_PLACEMENT_3D('',#88008,#55609,#55610);
#44651=AXIS2_PLACEMENT_3D('',#88009,#55611,#55612);
#44652=AXIS2_PLACEMENT_3D('',#88010,#55613,#55614);
#44653=AXIS2_PLACEMENT_3D('',#88011,#55615,#55616);
#44654=AXIS2_PLACEMENT_3D('',#88012,#55617,#55618);
#44655=AXIS2_PLACEMENT_3D('',#88013,#55619,#55620);
#44656=AXIS2_PLACEMENT_3D('',#88014,#55621,#55622);
#44657=AXIS2_PLACEMENT_3D('',#88017,#55623,#55624);
#44658=AXIS2_PLACEMENT_3D('',#88028,#55627,#55628);
#44659=AXIS2_PLACEMENT_3D('',#88032,#55630,#55631);
#44660=AXIS2_PLACEMENT_3D('',#88034,#55633,#55634);
#44661=AXIS2_PLACEMENT_3D('',#88035,#55635,#55636);
#44662=AXIS2_PLACEMENT_3D('',#88036,#55637,#55638);
#44663=AXIS2_PLACEMENT_3D('',#88037,#55639,#55640);
#44664=AXIS2_PLACEMENT_3D('',#88038,#55641,#55642);
#44665=AXIS2_PLACEMENT_3D('',#88039,#55643,#55644);
#44666=AXIS2_PLACEMENT_3D('',#88040,#55645,#55646);
#44667=AXIS2_PLACEMENT_3D('',#88043,#55647,#55648);
#44668=AXIS2_PLACEMENT_3D('',#88054,#55651,#55652);
#44669=AXIS2_PLACEMENT_3D('',#88058,#55654,#55655);
#44670=AXIS2_PLACEMENT_3D('',#88060,#55657,#55658);
#44671=AXIS2_PLACEMENT_3D('',#88061,#55659,#55660);
#44672=AXIS2_PLACEMENT_3D('',#88062,#55661,#55662);
#44673=AXIS2_PLACEMENT_3D('',#88063,#55663,#55664);
#44674=AXIS2_PLACEMENT_3D('',#88064,#55665,#55666);
#44675=AXIS2_PLACEMENT_3D('',#88065,#55667,#55668);
#44676=AXIS2_PLACEMENT_3D('',#88066,#55669,#55670);
#44677=AXIS2_PLACEMENT_3D('',#88069,#55671,#55672);
#44678=AXIS2_PLACEMENT_3D('',#88080,#55675,#55676);
#44679=AXIS2_PLACEMENT_3D('',#88084,#55678,#55679);
#44680=AXIS2_PLACEMENT_3D('',#88086,#55681,#55682);
#44681=AXIS2_PLACEMENT_3D('',#88087,#55683,#55684);
#44682=AXIS2_PLACEMENT_3D('',#88088,#55685,#55686);
#44683=AXIS2_PLACEMENT_3D('',#88089,#55687,#55688);
#44684=AXIS2_PLACEMENT_3D('',#88090,#55689,#55690);
#44685=AXIS2_PLACEMENT_3D('',#88091,#55691,#55692);
#44686=AXIS2_PLACEMENT_3D('',#88092,#55693,#55694);
#44687=AXIS2_PLACEMENT_3D('',#88095,#55695,#55696);
#44688=AXIS2_PLACEMENT_3D('',#88106,#55699,#55700);
#44689=AXIS2_PLACEMENT_3D('',#88110,#55702,#55703);
#44690=AXIS2_PLACEMENT_3D('',#88112,#55705,#55706);
#44691=AXIS2_PLACEMENT_3D('',#88113,#55707,#55708);
#44692=AXIS2_PLACEMENT_3D('',#88114,#55709,#55710);
#44693=AXIS2_PLACEMENT_3D('',#88115,#55711,#55712);
#44694=AXIS2_PLACEMENT_3D('',#88116,#55713,#55714);
#44695=AXIS2_PLACEMENT_3D('',#88117,#55715,#55716);
#44696=AXIS2_PLACEMENT_3D('',#88118,#55717,#55718);
#44697=AXIS2_PLACEMENT_3D('',#88121,#55719,#55720);
#44698=AXIS2_PLACEMENT_3D('',#88132,#55723,#55724);
#44699=AXIS2_PLACEMENT_3D('',#88136,#55726,#55727);
#44700=AXIS2_PLACEMENT_3D('',#88138,#55729,#55730);
#44701=AXIS2_PLACEMENT_3D('',#88139,#55731,#55732);
#44702=AXIS2_PLACEMENT_3D('',#88140,#55733,#55734);
#44703=AXIS2_PLACEMENT_3D('',#88141,#55735,#55736);
#44704=AXIS2_PLACEMENT_3D('',#88142,#55737,#55738);
#44705=AXIS2_PLACEMENT_3D('',#88143,#55739,#55740);
#44706=AXIS2_PLACEMENT_3D('',#88144,#55741,#55742);
#44707=AXIS2_PLACEMENT_3D('',#88147,#55743,#55744);
#44708=AXIS2_PLACEMENT_3D('',#88158,#55747,#55748);
#44709=AXIS2_PLACEMENT_3D('',#88162,#55750,#55751);
#44710=AXIS2_PLACEMENT_3D('',#88164,#55753,#55754);
#44711=AXIS2_PLACEMENT_3D('',#88165,#55755,#55756);
#44712=AXIS2_PLACEMENT_3D('',#88166,#55757,#55758);
#44713=AXIS2_PLACEMENT_3D('',#88167,#55759,#55760);
#44714=AXIS2_PLACEMENT_3D('',#88168,#55761,#55762);
#44715=AXIS2_PLACEMENT_3D('',#88169,#55763,#55764);
#44716=AXIS2_PLACEMENT_3D('',#88170,#55765,#55766);
#44717=AXIS2_PLACEMENT_3D('',#88173,#55767,#55768);
#44718=AXIS2_PLACEMENT_3D('',#88184,#55771,#55772);
#44719=AXIS2_PLACEMENT_3D('',#88188,#55774,#55775);
#44720=AXIS2_PLACEMENT_3D('',#88190,#55777,#55778);
#44721=AXIS2_PLACEMENT_3D('',#88191,#55779,#55780);
#44722=AXIS2_PLACEMENT_3D('',#88192,#55781,#55782);
#44723=AXIS2_PLACEMENT_3D('',#88193,#55783,#55784);
#44724=AXIS2_PLACEMENT_3D('',#88194,#55785,#55786);
#44725=AXIS2_PLACEMENT_3D('',#88195,#55787,#55788);
#44726=AXIS2_PLACEMENT_3D('',#88196,#55789,#55790);
#44727=AXIS2_PLACEMENT_3D('',#88199,#55791,#55792);
#44728=AXIS2_PLACEMENT_3D('',#88210,#55795,#55796);
#44729=AXIS2_PLACEMENT_3D('',#88214,#55798,#55799);
#44730=AXIS2_PLACEMENT_3D('',#88216,#55801,#55802);
#44731=AXIS2_PLACEMENT_3D('',#88217,#55803,#55804);
#44732=AXIS2_PLACEMENT_3D('',#88218,#55805,#55806);
#44733=AXIS2_PLACEMENT_3D('',#88219,#55807,#55808);
#44734=AXIS2_PLACEMENT_3D('',#88220,#55809,#55810);
#44735=AXIS2_PLACEMENT_3D('',#88221,#55811,#55812);
#44736=AXIS2_PLACEMENT_3D('',#88222,#55813,#55814);
#44737=AXIS2_PLACEMENT_3D('',#88225,#55815,#55816);
#44738=AXIS2_PLACEMENT_3D('',#88236,#55819,#55820);
#44739=AXIS2_PLACEMENT_3D('',#88240,#55822,#55823);
#44740=AXIS2_PLACEMENT_3D('',#88242,#55825,#55826);
#44741=AXIS2_PLACEMENT_3D('',#88243,#55827,#55828);
#44742=AXIS2_PLACEMENT_3D('',#88244,#55829,#55830);
#44743=AXIS2_PLACEMENT_3D('',#88245,#55831,#55832);
#44744=AXIS2_PLACEMENT_3D('',#88246,#55833,#55834);
#44745=AXIS2_PLACEMENT_3D('',#88247,#55835,#55836);
#44746=AXIS2_PLACEMENT_3D('',#88248,#55837,#55838);
#44747=AXIS2_PLACEMENT_3D('',#88251,#55839,#55840);
#44748=AXIS2_PLACEMENT_3D('',#88262,#55843,#55844);
#44749=AXIS2_PLACEMENT_3D('',#88266,#55846,#55847);
#44750=AXIS2_PLACEMENT_3D('',#88268,#55849,#55850);
#44751=AXIS2_PLACEMENT_3D('',#88269,#55851,#55852);
#44752=AXIS2_PLACEMENT_3D('',#88270,#55853,#55854);
#44753=AXIS2_PLACEMENT_3D('',#88271,#55855,#55856);
#44754=AXIS2_PLACEMENT_3D('',#88272,#55857,#55858);
#44755=AXIS2_PLACEMENT_3D('',#88273,#55859,#55860);
#44756=AXIS2_PLACEMENT_3D('',#88276,#55861,#55862);
#44757=AXIS2_PLACEMENT_3D('',#88287,#55865,#55866);
#44758=AXIS2_PLACEMENT_3D('',#88291,#55868,#55869);
#44759=AXIS2_PLACEMENT_3D('',#88293,#55871,#55872);
#44760=AXIS2_PLACEMENT_3D('',#88294,#55873,#55874);
#44761=AXIS2_PLACEMENT_3D('',#88295,#55875,#55876);
#44762=AXIS2_PLACEMENT_3D('',#88296,#55877,#55878);
#44763=AXIS2_PLACEMENT_3D('',#88297,#55879,#55880);
#44764=AXIS2_PLACEMENT_3D('',#88299,#55881,#55882);
#44765=AXIS2_PLACEMENT_3D('',#88301,#55883,#55884);
#44766=AXIS2_PLACEMENT_3D('',#88303,#55885,#55886);
#44767=AXIS2_PLACEMENT_3D('',#88304,#55887,#55888);
#44768=AXIS2_PLACEMENT_3D('',#88305,#55889,#55890);
#44769=AXIS2_PLACEMENT_3D('',#88306,#55891,#55892);
#44770=AXIS2_PLACEMENT_3D('',#88307,#55893,#55894);
#44771=AXIS2_PLACEMENT_3D('',#88308,#55895,#55896);
#44772=AXIS2_PLACEMENT_3D('',#88335,#55923,#55924);
#44773=AXIS2_PLACEMENT_3D('',#88337,#55926,#55927);
#44774=AXIS2_PLACEMENT_3D('',#88338,#55928,#55929);
#44775=AXIS2_PLACEMENT_3D('',#88339,#55930,#55931);
#44776=AXIS2_PLACEMENT_3D('',#88340,#55932,#55933);
#44777=AXIS2_PLACEMENT_3D('',#88341,#55934,#55935);
#44778=AXIS2_PLACEMENT_3D('',#88342,#55936,#55937);
#44779=AXIS2_PLACEMENT_3D('',#88343,#55938,#55939);
#44780=AXIS2_PLACEMENT_3D('',#88344,#55940,#55941);
#44781=AXIS2_PLACEMENT_3D('',#88345,#55942,#55943);
#44782=AXIS2_PLACEMENT_3D('',#88346,#55944,#55945);
#44783=AXIS2_PLACEMENT_3D('',#88347,#55946,#55947);
#44784=AXIS2_PLACEMENT_3D('',#88348,#55948,#55949);
#44785=AXIS2_PLACEMENT_3D('',#88349,#55950,#55951);
#44786=AXIS2_PLACEMENT_3D('',#88350,#55952,#55953);
#44787=AXIS2_PLACEMENT_3D('',#88351,#55954,#55955);
#44788=AXIS2_PLACEMENT_3D('',#88352,#55956,#55957);
#44789=AXIS2_PLACEMENT_3D('',#88353,#55958,#55959);
#44790=AXIS2_PLACEMENT_3D('',#88354,#55960,#55961);
#44791=AXIS2_PLACEMENT_3D('',#88355,#55962,#55963);
#44792=AXIS2_PLACEMENT_3D('',#88356,#55964,#55965);
#44793=AXIS2_PLACEMENT_3D('',#88357,#55966,#55967);
#44794=AXIS2_PLACEMENT_3D('',#88358,#55968,#55969);
#44795=AXIS2_PLACEMENT_3D('',#88359,#55970,#55971);
#44796=AXIS2_PLACEMENT_3D('',#88360,#55972,#55973);
#44797=AXIS2_PLACEMENT_3D('',#88361,#55974,#55975);
#44798=AXIS2_PLACEMENT_3D('',#88362,#55976,#55977);
#44799=AXIS2_PLACEMENT_3D('',#88363,#55978,#55979);
#44800=AXIS2_PLACEMENT_3D('',#88364,#55980,#55981);
#44801=AXIS2_PLACEMENT_3D('',#88365,#55982,#55983);
#44802=AXIS2_PLACEMENT_3D('',#88366,#55984,#55985);
#44803=AXIS2_PLACEMENT_3D('',#88367,#55986,#55987);
#44804=AXIS2_PLACEMENT_3D('',#88368,#55988,#55989);
#44805=AXIS2_PLACEMENT_3D('',#88369,#55990,#55991);
#44806=AXIS2_PLACEMENT_3D('',#88370,#55992,#55993);
#44807=AXIS2_PLACEMENT_3D('',#88371,#55994,#55995);
#44808=AXIS2_PLACEMENT_3D('',#88373,#55997,#55998);
#54726=DIRECTION('axis',(0.,0.,1.));
#54727=DIRECTION('refdir',(1.,0.,0.));
#54728=DIRECTION('center_axis',(1.,0.,0.));
#54729=DIRECTION('ref_axis',(0.,0.,-1.));
#54730=DIRECTION('center_axis',(-1.,0.,0.));
#54731=DIRECTION('ref_axis',(0.,-1.,1.83697019872103E-16));
#54732=DIRECTION('center_axis',(0.,-1.,-1.22464679914735E-16));
#54733=DIRECTION('ref_axis',(0.,-1.22464679914735E-16,1.));
#54734=DIRECTION('center_axis',(1.,0.,0.));
#54735=DIRECTION('ref_axis',(0.,-1.,1.83697019872103E-16));
#54736=DIRECTION('center_axis',(1.,0.,0.));
#54737=DIRECTION('ref_axis',(0.,-1.,1.83697019872103E-16));
#54738=DIRECTION('center_axis',(1.,0.,0.));
#54739=DIRECTION('ref_axis',(0.,1.,0.));
#54740=DIRECTION('',(-1.,0.,0.));
#54741=DIRECTION('center_axis',(1.,0.,0.));
#54742=DIRECTION('ref_axis',(0.,0.,-1.));
#54743=DIRECTION('center_axis',(1.,0.,0.));
#54744=DIRECTION('ref_axis',(0.,0.,-1.));
#54745=DIRECTION('center_axis',(1.,0.,0.));
#54746=DIRECTION('ref_axis',(0.,0.,-1.));
#54747=DIRECTION('center_axis',(1.,0.,0.));
#54748=DIRECTION('ref_axis',(0.,0.,-1.));
#54749=DIRECTION('center_axis',(-1.,0.,0.));
#54750=DIRECTION('ref_axis',(0.,-1.,1.83697019872103E-16));
#54751=DIRECTION('center_axis',(0.,-1.,-1.22464679914735E-16));
#54752=DIRECTION('ref_axis',(0.,-1.22464679914735E-16,1.));
#54753=DIRECTION('center_axis',(1.,0.,0.));
#54754=DIRECTION('ref_axis',(0.,-1.,1.83697019872103E-16));
#54755=DIRECTION('center_axis',(1.,0.,0.));
#54756=DIRECTION('ref_axis',(0.,-1.,1.83697019872103E-16));
#54757=DIRECTION('center_axis',(1.,0.,0.));
#54758=DIRECTION('ref_axis',(0.,1.,0.));
#54759=DIRECTION('',(-1.,0.,0.));
#54760=DIRECTION('center_axis',(1.,0.,0.));
#54761=DIRECTION('ref_axis',(0.,0.,-1.));
#54762=DIRECTION('center_axis',(1.,0.,0.));
#54763=DIRECTION('ref_axis',(0.,0.,-1.));
#54764=DIRECTION('center_axis',(1.,0.,0.));
#54765=DIRECTION('ref_axis',(0.,0.,-1.));
#54766=DIRECTION('center_axis',(-1.,0.,0.));
#54767=DIRECTION('ref_axis',(0.,-1.,1.83697019872103E-16));
#54768=DIRECTION('center_axis',(0.,-1.,-1.22464679914735E-16));
#54769=DIRECTION('ref_axis',(0.,-1.22464679914735E-16,1.));
#54770=DIRECTION('center_axis',(1.,0.,0.));
#54771=DIRECTION('ref_axis',(0.,-1.,3.06161699786838E-17));
#54772=DIRECTION('center_axis',(1.,0.,0.));
#54773=DIRECTION('ref_axis',(0.,-1.,3.06161699786838E-17));
#54774=DIRECTION('center_axis',(-1.,0.,0.));
#54775=DIRECTION('ref_axis',(0.,1.,0.));
#54776=DIRECTION('',(-0.998752338877845,-0.0499376169438921,-6.1155942747384E-18));
#54777=DIRECTION('center_axis',(1.,0.,0.));
#54778=DIRECTION('ref_axis',(0.,0.,-1.));
#54779=DIRECTION('center_axis',(1.,0.,0.));
#54780=DIRECTION('ref_axis',(0.,0.,-1.));
#54781=DIRECTION('center_axis',(1.,0.,0.));
#54782=DIRECTION('ref_axis',(0.,0.,-1.));
#54783=DIRECTION('center_axis',(-1.,0.,0.));
#54784=DIRECTION('ref_axis',(0.,-1.,3.06161699786838E-17));
#54785=DIRECTION('center_axis',(-1.,0.,0.));
#54786=DIRECTION('ref_axis',(0.,-1.,3.06161699786838E-17));
#54787=DIRECTION('center_axis',(0.,-1.,-1.22464679914735E-16));
#54788=DIRECTION('ref_axis',(0.,-1.22464679914735E-16,1.));
#54789=DIRECTION('center_axis',(1.,0.,0.));
#54790=DIRECTION('ref_axis',(0.,-1.,1.83697019872103E-16));
#54791=DIRECTION('center_axis',(1.,0.,0.));
#54792=DIRECTION('ref_axis',(0.,-1.,1.83697019872103E-16));
#54793=DIRECTION('center_axis',(1.,0.,0.));
#54794=DIRECTION('ref_axis',(0.,1.,0.));
#54795=DIRECTION('',(-1.,0.,0.));
#54796=DIRECTION('center_axis',(-1.,0.,0.));
#54797=DIRECTION('ref_axis',(0.,-1.,1.83697019872103E-16));
#54798=DIRECTION('center_axis',(-1.,0.,0.));
#54799=DIRECTION('ref_axis',(0.,-1.,1.83697019872103E-16));
#54800=DIRECTION('center_axis',(-1.,0.,0.));
#54801=DIRECTION('ref_axis',(0.,1.,0.));
#54802=DIRECTION('center_axis',(1.,0.,0.));
#54803=DIRECTION('ref_axis',(0.,0.,-1.));
#54804=DIRECTION('center_axis',(1.,0.,0.));
#54805=DIRECTION('ref_axis',(0.,0.,-1.));
#54806=DIRECTION('center_axis',(1.,0.,0.));
#54807=DIRECTION('ref_axis',(0.,0.,-1.));
#54808=DIRECTION('center_axis',(1.,0.,0.));
#54809=DIRECTION('ref_axis',(0.,0.,-1.));
#54810=DIRECTION('center_axis',(1.,0.,0.));
#54811=DIRECTION('ref_axis',(0.,0.,-1.));
#54812=DIRECTION('center_axis',(1.,0.,0.));
#54813=DIRECTION('ref_axis',(0.,0.,-1.));
#54814=DIRECTION('',(-0.707106781186553,-0.707106781186542,-8.65956056235487E-17));
#54815=DIRECTION('center_axis',(1.,0.,0.));
#54816=DIRECTION('ref_axis',(0.,0.,-1.));
#54817=DIRECTION('center_axis',(1.,0.,0.));
#54818=DIRECTION('ref_axis',(0.,0.,-1.));
#54819=DIRECTION('center_axis',(0.,-1.,-1.22464679914735E-16));
#54820=DIRECTION('ref_axis',(0.,-1.22464679914735E-16,1.));
#54821=DIRECTION('center_axis',(1.,0.,0.));
#54822=DIRECTION('ref_axis',(0.,-1.,3.06161699786838E-17));
#54823=DIRECTION('center_axis',(1.,0.,0.));
#54824=DIRECTION('ref_axis',(0.,-1.,3.06161699786838E-17));
#54825=DIRECTION('center_axis',(1.,0.,0.));
#54826=DIRECTION('ref_axis',(0.,1.,0.));
#54827=DIRECTION('',(-0.707106781186563,0.707106781186532,8.65956056235474E-17));
#54828=DIRECTION('center_axis',(-1.,0.,0.));
#54829=DIRECTION('ref_axis',(0.,-1.,3.06161699786838E-17));
#54830=DIRECTION('center_axis',(-1.,0.,0.));
#54831=DIRECTION('ref_axis',(0.,-1.,3.06161699786838E-17));
#54832=DIRECTION('center_axis',(-1.,0.,0.));
#54833=DIRECTION('ref_axis',(0.,-0.813895208686417,-0.581011694613193));
#54834=DIRECTION('center_axis',(1.,0.,0.));
#54835=DIRECTION('ref_axis',(0.,-0.999953846953934,0.00960749509648641));
#54836=DIRECTION('',(1.,0.,0.));
#54837=DIRECTION('center_axis',(1.,0.,0.));
#54838=DIRECTION('ref_axis',(0.,-0.813895208686417,-0.581011694613193));
#54839=DIRECTION('',(-1.,0.,0.));
#54840=DIRECTION('center_axis',(1.,0.,0.));
#54841=DIRECTION('ref_axis',(0.,-0.499999999999999,0.866025403784439));
#54842=DIRECTION('center_axis',(-2.22034356890148E-15,0.00960749509648415,
0.999953846953934));
#54843=DIRECTION('ref_axis',(-1.,0.,-2.22044604925028E-15));
#54844=DIRECTION('center_axis',(1.,0.,0.));
#54845=DIRECTION('ref_axis',(0.,-0.5,0.866025403784439));
#54846=DIRECTION('center_axis',(-1.48763331779908E-14,-0.870789181622326,
0.491656588656675));
#54847=DIRECTION('ref_axis',(0.,0.491656588656675,0.870789181622326));
#54848=DIRECTION('center_axis',(-1.,0.,0.));
#54849=DIRECTION('ref_axis',(0.,-0.5,0.866025403784439));
#54850=DIRECTION('center_axis',(0.,0.,1.));
#54851=DIRECTION('ref_axis',(1.,0.,0.));
#54852=DIRECTION('center_axis',(0.,-0.94884262159901,0.315749393407364));
#54853=DIRECTION('ref_axis',(0.,0.315749393407364,0.94884262159901));
#54854=DIRECTION('center_axis',(1.,0.,0.));
#54855=DIRECTION('ref_axis',(0.,0.910118491774079,0.41434807943428));
#54856=DIRECTION('center_axis',(1.,0.,0.));
#54857=DIRECTION('ref_axis',(0.,0.97959651120185,-0.200974314879201));
#54858=DIRECTION('',(1.,0.,0.));
#54859=DIRECTION('center_axis',(1.,0.,0.));
#54860=DIRECTION('ref_axis',(0.,0.910118491774079,0.41434807943428));
#54861=DIRECTION('',(-1.,0.,0.));
#54862=DIRECTION('center_axis',(0.,0.,1.));
#54863=DIRECTION('ref_axis',(1.,0.,0.));
#54864=DIRECTION('center_axis',(0.,0.200974314879202,0.97959651120185));
#54865=DIRECTION('ref_axis',(0.,-0.97959651120185,0.200974314879202));
#54866=DIRECTION('center_axis',(1.,0.,0.));
#54867=DIRECTION('ref_axis',(0.,1.,0.));
#54868=DIRECTION('center_axis',(1.,0.,0.));
#54869=DIRECTION('ref_axis',(0.,0.475007952993551,0.879981502415179));
#54870=DIRECTION('',(-1.,0.,0.));
#54871=DIRECTION('center_axis',(1.,0.,0.));
#54872=DIRECTION('ref_axis',(0.,0.,-1.));
#54873=DIRECTION('center_axis',(1.,0.,0.));
#54874=DIRECTION('ref_axis',(0.,0.,-1.));
#54875=DIRECTION('center_axis',(-1.,0.,0.));
#54876=DIRECTION('ref_axis',(0.,0.475007952993551,0.879981502415179));
#54877=DIRECTION('center_axis',(0.,-0.74786830671981,0.663847117794485));
#54878=DIRECTION('ref_axis',(-1.,0.,0.));
#54879=DIRECTION('center_axis',(-1.,0.,0.));
#54880=DIRECTION('ref_axis',(0.,0.,1.));
#54881=DIRECTION('center_axis',(1.,0.,0.));
#54882=DIRECTION('ref_axis',(0.,-1.,1.83697019872103E-16));
#54883=DIRECTION('center_axis',(-1.,0.,0.));
#54884=DIRECTION('ref_axis',(0.,-0.999590312448718,0.0286217969155305));
#54885=DIRECTION('center_axis',(-1.,0.,0.));
#54886=DIRECTION('ref_axis',(0.,-0.520505045907276,-0.853858593202097));
#54887=DIRECTION('center_axis',(-1.,0.,0.));
#54888=DIRECTION('ref_axis',(0.,0.517748535001257,-0.855532848290498));
#54889=DIRECTION('center_axis',(-1.,0.,0.));
#54890=DIRECTION('ref_axis',(0.,0.999445904365848,0.0332848951678069));
#54891=DIRECTION('center_axis',(1.,0.,0.));
#54892=DIRECTION('ref_axis',(0.,0.,-1.));
#54893=DIRECTION('center_axis',(1.,0.,0.));
#54894=DIRECTION('ref_axis',(0.,-0.999590312448718,0.0286217969155305));
#54895=DIRECTION('center_axis',(-4.46252623474304E-16,-0.200974314879201,
0.97959651120185));
#54896=DIRECTION('ref_axis',(0.,0.97959651120185,0.200974314879201));
#54897=DIRECTION('center_axis',(1.,0.,0.));
#54898=DIRECTION('ref_axis',(0.,-1.,1.22464679914735E-16));
#54899=DIRECTION('center_axis',(1.,0.,0.));
#54900=DIRECTION('ref_axis',(0.,0.,-1.));
#54901=DIRECTION('',(1.,0.,0.));
#54902=DIRECTION('center_axis',(1.,0.,0.));
#54903=DIRECTION('ref_axis',(0.,-0.0962232830876605,-0.995359774047471));
#54904=DIRECTION('center_axis',(1.,0.,0.));
#54905=DIRECTION('ref_axis',(0.,-0.663847117794486,-0.747868306719809));
#54906=DIRECTION('',(1.,0.,0.));
#54907=DIRECTION('center_axis',(1.,0.,0.));
#54908=DIRECTION('ref_axis',(0.,-0.0962232830876605,-0.995359774047471));
#54909=DIRECTION('center_axis',(0.0431948626350049,-0.996646165621364,0.0695026934310885));
#54910=DIRECTION('ref_axis',(-0.526079934143921,-0.0818316598403858,-0.846488914480807));
#54911=DIRECTION('center_axis',(0.,-0.86118168652584,-0.508297258297258));
#54912=DIRECTION('ref_axis',(0.,-0.508297258297258,0.86118168652584));
#54913=DIRECTION('center_axis',(1.,0.,0.));
#54914=DIRECTION('ref_axis',(0.,1.,1.83697019872103E-16));
#54915=DIRECTION('center_axis',(1.,0.,0.));
#54916=DIRECTION('ref_axis',(0.,0.999445904365848,0.0332848951678069));
#54917=DIRECTION('',(-1.,0.,0.));
#54918=DIRECTION('center_axis',(1.,0.,0.));
#54919=DIRECTION('ref_axis',(0.,0.,-1.));
#54920=DIRECTION('center_axis',(1.,0.,0.));
#54921=DIRECTION('ref_axis',(0.,1.,1.83697019872103E-16));
#54922=DIRECTION('center_axis',(-1.12864663903091E-15,0.861181686525838,
-0.508297258297262));
#54923=DIRECTION('ref_axis',(-1.,0.,2.22044604925028E-15));
#54924=DIRECTION('center_axis',(1.,0.,0.));
#54925=DIRECTION('ref_axis',(0.,0.,-1.));
#54926=DIRECTION('center_axis',(0.,-1.,-1.22464679914735E-16));
#54927=DIRECTION('ref_axis',(0.,-1.22464679914735E-16,1.));
#54928=DIRECTION('center_axis',(-1.,0.,0.));
#54929=DIRECTION('ref_axis',(0.,-0.983415102160779,-0.181369062527503));
#54930=DIRECTION('',(1.,0.,0.));
#54931=DIRECTION('',(-1.,0.,0.));
#54932=DIRECTION('center_axis',(0.,1.,0.));
#54933=DIRECTION('ref_axis',(-1.,0.,0.));
#54934=DIRECTION('',(0.,0.,1.));
#54935=DIRECTION('',(1.,0.,0.));
#54936=DIRECTION('',(0.,0.,1.));
#54937=DIRECTION('center_axis',(1.,0.,0.));
#54938=DIRECTION('ref_axis',(0.,-0.983415102160779,0.181369062527503));
#54939=DIRECTION('',(-1.,0.,0.));
#54940=DIRECTION('center_axis',(-1.,0.,0.));
#54941=DIRECTION('ref_axis',(0.,0.910118491774079,-0.414348079434279));
#54942=DIRECTION('center_axis',(1.,0.,0.));
#54943=DIRECTION('ref_axis',(0.,0.491656588656675,-0.870789181622327));
#54944=DIRECTION('center_axis',(1.,0.,0.));
#54945=DIRECTION('ref_axis',(0.,0.910118491774079,-0.414348079434279));
#54946=DIRECTION('',(-1.,0.,0.));
#54947=DIRECTION('center_axis',(0.,0.,1.));
#54948=DIRECTION('ref_axis',(1.,0.,0.));
#54949=DIRECTION('center_axis',(0.,0.870789181622326,0.491656588656675));
#54950=DIRECTION('ref_axis',(0.,-0.491656588656675,0.870789181622327));
#54951=DIRECTION('center_axis',(1.,0.,0.));
#54952=DIRECTION('ref_axis',(0.,0.,-1.));
#54953=DIRECTION('center_axis',(1.,0.,0.));
#54954=DIRECTION('ref_axis',(0.,-0.520505045907276,-0.853858593202097));
#54955=DIRECTION('center_axis',(0.,0.00960749509648418,-0.999953846953934));
#54956=DIRECTION('ref_axis',(0.,-0.999953846953934,-0.00960749509648418));
#54957=DIRECTION('center_axis',(1.,0.,0.));
#54958=DIRECTION('ref_axis',(0.,-0.500000000000001,-0.866025403784438));
#54959=DIRECTION('center_axis',(1.,0.,0.));
#54960=DIRECTION('ref_axis',(0.,-0.866025403784438,0.5));
#54961=DIRECTION('',(1.,0.,0.));
#54962=DIRECTION('center_axis',(-1.,0.,0.));
#54963=DIRECTION('ref_axis',(0.,-0.0962232830876605,0.995359774047471));
#54964=DIRECTION('center_axis',(1.,0.,0.));
#54965=DIRECTION('ref_axis',(0.,0.508297258297259,0.861181686525839));
#54966=DIRECTION('',(1.,0.,0.));
#54967=DIRECTION('center_axis',(1.,0.,0.));
#54968=DIRECTION('ref_axis',(0.,-0.0962232830876605,0.995359774047471));
#54969=DIRECTION('center_axis',(0.0431948626350049,-0.996646165621364,-0.0695026934310867));
#54970=DIRECTION('ref_axis',(-0.526079934143921,-0.0818316598403823,0.846488914480808));
#54971=DIRECTION('center_axis',(0.,0.747868306719809,0.663847117794486));
#54972=DIRECTION('ref_axis',(0.,0.663847117794486,-0.747868306719809));
#54973=DIRECTION('center_axis',(1.,0.,0.));
#54974=DIRECTION('ref_axis',(0.,0.,-1.));
#54975=DIRECTION('center_axis',(0.,0.94884262159901,0.315749393407364));
#54976=DIRECTION('ref_axis',(-1.,0.,0.));
#54977=DIRECTION('center_axis',(1.,0.,0.));
#54978=DIRECTION('ref_axis',(0.,0.517748535001257,-0.855532848290498));
#54979=DIRECTION('center_axis',(0.,0.,1.));
#54980=DIRECTION('ref_axis',(1.,0.,0.));
#54981=DIRECTION('center_axis',(-1.,0.,0.));
#54982=DIRECTION('ref_axis',(0.,-0.813895208686417,0.581011694613192));
#54983=DIRECTION('center_axis',(1.,0.,0.));
#54984=DIRECTION('ref_axis',(0.,1.,0.));
#54985=DIRECTION('',(-1.,0.,0.));
#54986=DIRECTION('center_axis',(1.,0.,0.));
#54987=DIRECTION('ref_axis',(0.,0.,-1.));
#54988=DIRECTION('center_axis',(1.,0.,0.));
#54989=DIRECTION('ref_axis',(0.,-0.813895208686417,0.581011694613193));
#54990=DIRECTION('center_axis',(1.,0.,0.));
#54991=DIRECTION('ref_axis',(0.,-0.813895208686417,0.581011694613193));
#54992=DIRECTION('center_axis',(1.,0.,0.));
#54993=DIRECTION('ref_axis',(0.,0.,-1.));
#54994=DIRECTION('center_axis',(1.,0.,0.));
#54995=DIRECTION('ref_axis',(0.,-1.,1.22464679914735E-16));
#54996=DIRECTION('center_axis',(1.,0.,0.));
#54997=DIRECTION('ref_axis',(0.,0.,-1.));
#54998=DIRECTION('center_axis',(1.,0.,0.));
#54999=DIRECTION('ref_axis',(0.,0.,-1.));
#55000=DIRECTION('center_axis',(1.,0.,0.));
#55001=DIRECTION('ref_axis',(0.,1.,0.));
#55002=DIRECTION('center_axis',(1.,0.,0.));
#55003=DIRECTION('ref_axis',(0.,1.,0.));
#55004=DIRECTION('center_axis',(1.,0.,0.));
#55005=DIRECTION('ref_axis',(0.,0.,-1.));
#55006=DIRECTION('',(1.,0.,0.));
#55007=DIRECTION('center_axis',(-1.,0.,0.));
#55008=DIRECTION('ref_axis',(0.,0.,1.));
#55009=DIRECTION('center_axis',(-1.,0.,0.));
#55010=DIRECTION('ref_axis',(0.,-1.,-1.22464679914735E-16));
#55011=DIRECTION('center_axis',(-1.,0.,0.));
#55012=DIRECTION('ref_axis',(0.,-1.,0.));
#55013=DIRECTION('center_axis',(-1.,0.,0.));
#55014=DIRECTION('ref_axis',(0.,0.,1.));
#55015=DIRECTION('center_axis',(-1.,0.,0.));
#55016=DIRECTION('ref_axis',(0.,0.5,-0.866025403784439));
#55017=DIRECTION('center_axis',(-1.,0.,0.));
#55018=DIRECTION('ref_axis',(0.,0.648777766689775,-0.760977929672752));
#55019=DIRECTION('',(-1.,0.,0.));
#55020=DIRECTION('',(1.,0.,0.));
#55021=DIRECTION('center_axis',(1.,0.,0.));
#55022=DIRECTION('ref_axis',(0.,0.334637335471004,-0.942346992200255));
#55023=DIRECTION('',(1.,0.,0.));
#55024=DIRECTION('',(-1.,0.,0.));
#55025=DIRECTION('center_axis',(1.,0.,0.));
#55026=DIRECTION('ref_axis',(0.,0.,-1.));
#55027=DIRECTION('center_axis',(1.,0.,0.));
#55028=DIRECTION('ref_axis',(0.,0.,-1.));
#55029=DIRECTION('center_axis',(1.,0.,0.));
#55030=DIRECTION('ref_axis',(0.,0.5,-0.866025403784439));
#55031=DIRECTION('center_axis',(0.,-0.5,0.866025403784439));
#55032=DIRECTION('ref_axis',(-1.,0.,0.));
#55033=DIRECTION('',(0.,-0.866025403784439,-0.5));
#55034=DIRECTION('',(0.,-0.866025403784439,-0.5));
#55035=DIRECTION('center_axis',(-1.,0.,0.));
#55036=DIRECTION('ref_axis',(0.,0.5,-0.866025403784439));
#55037=DIRECTION('center_axis',(1.,0.,0.));
#55038=DIRECTION('ref_axis',(0.,1.,0.));
#55039=DIRECTION('center_axis',(1.,0.,0.));
#55040=DIRECTION('ref_axis',(0.,0.,-1.));
#55041=DIRECTION('center_axis',(1.,0.,0.));
#55042=DIRECTION('ref_axis',(0.,1.,0.));
#55043=DIRECTION('',(-1.,0.,0.));
#55044=DIRECTION('center_axis',(1.,0.,0.));
#55045=DIRECTION('ref_axis',(0.,0.,-1.));
#55046=DIRECTION('center_axis',(-1.,0.,0.));
#55047=DIRECTION('ref_axis',(0.,0.,1.));
#55048=DIRECTION('center_axis',(-1.,0.,0.));
#55049=DIRECTION('ref_axis',(0.,0.5,0.866025403784438));
#55050=DIRECTION('center_axis',(-1.,0.,0.));
#55051=DIRECTION('ref_axis',(0.,0.334637335471004,0.942346992200255));
#55052=DIRECTION('',(-1.,0.,0.));
#55053=DIRECTION('center_axis',(1.,0.,0.));
#55054=DIRECTION('ref_axis',(0.,0.648777766689778,0.76097792967275));
#55055=DIRECTION('',(1.,0.,0.));
#55056=DIRECTION('center_axis',(1.,0.,0.));
#55057=DIRECTION('ref_axis',(0.,0.,-1.));
#55058=DIRECTION('center_axis',(1.,0.,0.));
#55059=DIRECTION('ref_axis',(0.,0.,-1.));
#55060=DIRECTION('center_axis',(1.,0.,0.));
#55061=DIRECTION('ref_axis',(0.,0.5,0.866025403784438));
#55062=DIRECTION('center_axis',(0.,-0.5,-0.866025403784438));
#55063=DIRECTION('ref_axis',(-1.,0.,0.));
#55064=DIRECTION('',(0.,0.866025403784438,-0.5));
#55065=DIRECTION('',(0.,0.866025403784438,-0.5));
#55066=DIRECTION('center_axis',(-1.,0.,0.));
#55067=DIRECTION('ref_axis',(0.,0.5,0.866025403784438));
#55068=DIRECTION('center_axis',(-1.,0.,0.));
#55069=DIRECTION('ref_axis',(0.,0.593489101493648,0.804842025746831));
#55070=DIRECTION('center_axis',(-1.,0.,0.));
#55071=DIRECTION('ref_axis',(0.,0.593489101493648,0.804842025746831));
#55072=DIRECTION('',(1.,0.,0.));
#55073=DIRECTION('center_axis',(-1.,0.,0.));
#55074=DIRECTION('ref_axis',(0.,0.593489101493648,0.804842025746831));
#55075=DIRECTION('',(1.,0.,0.));
#55076=DIRECTION('center_axis',(-1.,0.,0.));
#55077=DIRECTION('ref_axis',(0.,0.593489101493648,0.804842025746831));
#55078=DIRECTION('center_axis',(-1.,0.,0.));
#55079=DIRECTION('ref_axis',(0.,0.593489101493648,0.804842025746831));
#55080=DIRECTION('',(1.,0.,0.));
#55081=DIRECTION('center_axis',(1.,0.,0.));
#55082=DIRECTION('ref_axis',(0.,0.593489101493648,0.804842025746831));
#55083=DIRECTION('',(-1.,0.,0.));
#55084=DIRECTION('center_axis',(1.,0.,0.));
#55085=DIRECTION('ref_axis',(0.,1.,0.));
#55086=DIRECTION('center_axis',(1.,0.,0.));
#55087=DIRECTION('ref_axis',(0.,0.,-1.));
#55088=DIRECTION('center_axis',(1.,0.,0.));
#55089=DIRECTION('ref_axis',(0.,0.,-1.));
#55090=DIRECTION('center_axis',(1.,0.,0.));
#55091=DIRECTION('ref_axis',(0.,0.,-1.));
#55092=DIRECTION('center_axis',(0.,0.,1.));
#55093=DIRECTION('ref_axis',(0.,-1.,0.));
#55094=DIRECTION('',(0.,1.,0.));
#55095=DIRECTION('',(-1.,0.,0.));
#55096=DIRECTION('center_axis',(1.,0.,0.));
#55097=DIRECTION('ref_axis',(0.,0.,-1.));
#55098=DIRECTION('center_axis',(1.,0.,0.));
#55099=DIRECTION('ref_axis',(0.,0.,-1.));
#55100=DIRECTION('',(0.,-0.239315664287558,0.970941817426052));
#55101=DIRECTION('center_axis',(-1.,0.,0.));
#55102=DIRECTION('ref_axis',(0.,0.89953724027626,-0.436844083576932));
#55103=DIRECTION('center_axis',(1.,0.,0.));
#55104=DIRECTION('ref_axis',(0.,0.,-1.));
#55105=DIRECTION('center_axis',(-1.,0.,0.));
#55106=DIRECTION('ref_axis',(0.,0.89953724027626,-0.436844083576932));
#55107=DIRECTION('',(0.,-0.464723172043769,0.88545602565321));
#55108=DIRECTION('center_axis',(-1.,0.,0.));
#55109=DIRECTION('ref_axis',(0.,0.97794195496755,-0.208876836231895));
#55110=DIRECTION('center_axis',(1.,0.,0.));
#55111=DIRECTION('ref_axis',(0.,0.,-1.));
#55112=DIRECTION('center_axis',(-1.,0.,0.));
#55113=DIRECTION('ref_axis',(0.,0.97794195496755,-0.208876836231895));
#55114=DIRECTION('',(0.,-0.663122658240795,0.748510748171101));
#55115=DIRECTION('center_axis',(-1.,0.,0.));
#55116=DIRECTION('ref_axis',(0.,0.999512237910499,0.0312295735985313));
#55117=DIRECTION('center_axis',(1.,0.,0.));
#55118=DIRECTION('ref_axis',(0.,0.,-1.));
#55119=DIRECTION('center_axis',(-1.,0.,0.));
#55120=DIRECTION('ref_axis',(0.,0.999512237910499,0.0312295735985313));
#55121=DIRECTION('',(0.,-0.822983865893656,0.568064746731156));
#55122=DIRECTION('center_axis',(-1.,0.,0.));
#55123=DIRECTION('ref_axis',(0.,0.96299450266525,0.269521034126294));
#55124=DIRECTION('center_axis',(1.,0.,0.));
#55125=DIRECTION('ref_axis',(0.,0.,-1.));
#55126=DIRECTION('center_axis',(-1.,0.,0.));
#55127=DIRECTION('ref_axis',(0.,0.96299450266525,0.269521034126294));
#55128=DIRECTION('',(0.,-0.935016242685415,0.354604887042536));
#55129=DIRECTION('center_axis',(-1.,0.,0.));
#55130=DIRECTION('ref_axis',(0.,0.870511027267693,0.492148911819732));
#55131=DIRECTION('center_axis',(1.,0.,0.));
#55132=DIRECTION('ref_axis',(0.,0.,-1.));
#55133=DIRECTION('center_axis',(-1.,0.,0.));
#55134=DIRECTION('ref_axis',(0.,0.870511027267693,0.492148911819732));
#55135=DIRECTION('',(0.,-0.992708874098054,0.120536680255323));
#55136=DIRECTION('center_axis',(-1.,0.,0.));
#55137=DIRECTION('ref_axis',(0.,0.727436615144173,0.686174883646719));
#55138=DIRECTION('center_axis',(1.,0.,0.));
#55139=DIRECTION('ref_axis',(0.,0.,-1.));
#55140=DIRECTION('center_axis',(-1.,0.,0.));
#55141=DIRECTION('ref_axis',(0.,0.727436615144173,0.686174883646719));
#55142=DIRECTION('',(0.,-0.992708874098054,-0.120536680255323));
#55143=DIRECTION('center_axis',(-1.,0.,0.));
#55144=DIRECTION('ref_axis',(0.,0.542086231072989,0.840322865380374));
#55145=DIRECTION('center_axis',(1.,0.,0.));
#55146=DIRECTION('ref_axis',(0.,0.,-1.));
#55147=DIRECTION('center_axis',(-1.,0.,0.));
#55148=DIRECTION('ref_axis',(0.,0.542086231072989,0.840322865380374));
#55149=DIRECTION('',(0.,-0.935016242685415,-0.354604887042536));
#55150=DIRECTION('center_axis',(-1.,0.,0.));
#55151=DIRECTION('ref_axis',(0.,0.325231765655118,0.945634336627459));
#55152=DIRECTION('center_axis',(1.,0.,0.));
#55153=DIRECTION('ref_axis',(0.,0.,-1.));
#55154=DIRECTION('center_axis',(-1.,0.,0.));
#55155=DIRECTION('ref_axis',(0.,0.325231765655118,0.945634336627459));
#55156=DIRECTION('',(0.,-0.822983865893656,-0.568064746731156));
#55157=DIRECTION('center_axis',(-1.,0.,0.));
#55158=DIRECTION('ref_axis',(0.,0.0894760121867377,0.995988977470714));
#55159=DIRECTION('center_axis',(1.,0.,0.));
#55160=DIRECTION('ref_axis',(0.,0.,-1.));
#55161=DIRECTION('center_axis',(-1.,0.,0.));
#55162=DIRECTION('ref_axis',(0.,0.0894760121867377,0.995988977470714));
#55163=DIRECTION('',(0.,-0.663122658240796,-0.748510748171101));
#55164=DIRECTION('center_axis',(-1.,0.,0.));
#55165=DIRECTION('ref_axis',(0.,-0.151479761877859,0.988460359216002));
#55166=DIRECTION('center_axis',(1.,0.,0.));
#55167=DIRECTION('ref_axis',(0.,0.,-1.));
#55168=DIRECTION('center_axis',(-1.,0.,0.));
#55169=DIRECTION('ref_axis',(0.,-0.151479761877859,0.988460359216002));
#55170=DIRECTION('',(0.,-0.464723172043769,-0.88545602565321));
#55171=DIRECTION('center_axis',(-1.,0.,0.));
#55172=DIRECTION('ref_axis',(0.,-0.383632082788652,0.923486017790871));
#55173=DIRECTION('center_axis',(1.,0.,0.));
#55174=DIRECTION('ref_axis',(0.,0.,-1.));
#55175=DIRECTION('center_axis',(-1.,0.,0.));
#55176=DIRECTION('ref_axis',(0.,-0.383632082788652,0.923486017790871));
#55177=DIRECTION('',(0.,-0.239315664287558,-0.970941817426052));
#55178=DIRECTION('center_axis',(-1.,0.,0.));
#55179=DIRECTION('ref_axis',(0.,-0.593489101493646,0.804842025746833));
#55180=DIRECTION('center_axis',(1.,0.,0.));
#55181=DIRECTION('ref_axis',(0.,0.,-1.));
#55182=DIRECTION('center_axis',(-1.,0.,0.));
#55183=DIRECTION('ref_axis',(0.,-0.593489101493646,0.804842025746833));
#55184=DIRECTION('',(0.,-1.22464679914735E-16,-1.));
#55185=DIRECTION('center_axis',(-1.,0.,0.));
#55186=DIRECTION('ref_axis',(0.,-0.768854690864945,0.639423540648114));
#55187=DIRECTION('center_axis',(1.,0.,0.));
#55188=DIRECTION('ref_axis',(0.,0.,-1.));
#55189=DIRECTION('center_axis',(-1.,0.,0.));
#55190=DIRECTION('ref_axis',(0.,-0.768854690864945,0.639423540648114));
#55191=DIRECTION('',(0.,0.239315664287557,-0.970941817426052));
#55192=DIRECTION('center_axis',(-1.,0.,0.));
#55193=DIRECTION('ref_axis',(0.,-0.899537240276258,0.436844083576936));
#55194=DIRECTION('center_axis',(1.,0.,0.));
#55195=DIRECTION('ref_axis',(0.,0.,-1.));
#55196=DIRECTION('center_axis',(-1.,0.,0.));
#55197=DIRECTION('ref_axis',(0.,-0.899537240276258,0.436844083576936));
#55198=DIRECTION('',(0.,0.464723172043768,-0.88545602565321));
#55199=DIRECTION('center_axis',(-1.,0.,0.));
#55200=DIRECTION('ref_axis',(0.,-0.97794195496755,0.208876836231895));
#55201=DIRECTION('center_axis',(1.,0.,0.));
#55202=DIRECTION('ref_axis',(0.,0.,-1.));
#55203=DIRECTION('center_axis',(-1.,0.,0.));
#55204=DIRECTION('ref_axis',(0.,-0.97794195496755,0.208876836231895));
#55205=DIRECTION('',(0.,0.663122658240795,-0.748510748171101));
#55206=DIRECTION('center_axis',(-1.,0.,0.));
#55207=DIRECTION('ref_axis',(0.,-0.999512237910499,-0.0312295735985302));
#55208=DIRECTION('center_axis',(1.,0.,0.));
#55209=DIRECTION('ref_axis',(0.,0.,-1.));
#55210=DIRECTION('center_axis',(-1.,0.,0.));
#55211=DIRECTION('ref_axis',(0.,-0.999512237910499,-0.0312295735985302));
#55212=DIRECTION('',(0.,0.822983865893656,-0.568064746731156));
#55213=DIRECTION('center_axis',(-1.,0.,0.));
#55214=DIRECTION('ref_axis',(0.,-0.96299450266525,-0.269521034126296));
#55215=DIRECTION('center_axis',(1.,0.,0.));
#55216=DIRECTION('ref_axis',(0.,0.,-1.));
#55217=DIRECTION('center_axis',(-1.,0.,0.));
#55218=DIRECTION('ref_axis',(0.,-0.96299450266525,-0.269521034126296));
#55219=DIRECTION('',(0.,0.935016242685415,-0.354604887042536));
#55220=DIRECTION('center_axis',(-1.,0.,0.));
#55221=DIRECTION('ref_axis',(0.,-0.87051102726769,-0.492148911819736));
#55222=DIRECTION('center_axis',(1.,0.,0.));
#55223=DIRECTION('ref_axis',(0.,0.,-1.));
#55224=DIRECTION('center_axis',(-1.,0.,0.));
#55225=DIRECTION('ref_axis',(0.,-0.87051102726769,-0.492148911819736));
#55226=DIRECTION('',(0.,0.992708874098054,-0.120536680255324));
#55227=DIRECTION('center_axis',(-1.,0.,0.));
#55228=DIRECTION('ref_axis',(0.,-0.727436615144171,-0.686174883646721));
#55229=DIRECTION('center_axis',(1.,0.,0.));
#55230=DIRECTION('ref_axis',(0.,0.,-1.));
#55231=DIRECTION('center_axis',(-1.,0.,0.));
#55232=DIRECTION('ref_axis',(0.,-0.727436615144171,-0.686174883646721));
#55233=DIRECTION('',(0.,0.992708874098054,0.120536680255322));
#55234=DIRECTION('center_axis',(-1.,0.,0.));
#55235=DIRECTION('ref_axis',(0.,-0.542086231072992,-0.840322865380372));
#55236=DIRECTION('center_axis',(1.,0.,0.));
#55237=DIRECTION('ref_axis',(0.,0.,-1.));
#55238=DIRECTION('center_axis',(-1.,0.,0.));
#55239=DIRECTION('ref_axis',(0.,-0.542086231072992,-0.840322865380372));
#55240=DIRECTION('',(0.,0.935016242685415,0.354604887042536));
#55241=DIRECTION('center_axis',(-1.,0.,0.));
#55242=DIRECTION('ref_axis',(0.,-0.325231765655117,-0.945634336627459));
#55243=DIRECTION('center_axis',(1.,0.,0.));
#55244=DIRECTION('ref_axis',(0.,0.,-1.));
#55245=DIRECTION('center_axis',(-1.,0.,0.));
#55246=DIRECTION('ref_axis',(0.,-0.325231765655117,-0.945634336627459));
#55247=DIRECTION('',(0.,0.822983865893656,0.568064746731156));
#55248=DIRECTION('center_axis',(-1.,0.,0.));
#55249=DIRECTION('ref_axis',(0.,-0.0894760121867388,-0.995988977470714));
#55250=DIRECTION('center_axis',(1.,0.,0.));
#55251=DIRECTION('ref_axis',(0.,0.,-1.));
#55252=DIRECTION('center_axis',(-1.,0.,0.));
#55253=DIRECTION('ref_axis',(0.,-0.0894760121867388,-0.995988977470714));
#55254=DIRECTION('',(0.,0.663122658240796,0.748510748171101));
#55255=DIRECTION('center_axis',(-1.,0.,0.));
#55256=DIRECTION('ref_axis',(0.,0.151479761877861,-0.988460359216002));
#55257=DIRECTION('center_axis',(1.,0.,0.));
#55258=DIRECTION('ref_axis',(0.,0.,-1.));
#55259=DIRECTION('center_axis',(-1.,0.,0.));
#55260=DIRECTION('ref_axis',(0.,0.151479761877861,-0.988460359216002));
#55261=DIRECTION('',(0.,0.464723172043769,0.88545602565321));
#55262=DIRECTION('center_axis',(-1.,0.,0.));
#55263=DIRECTION('ref_axis',(0.,0.383632082788654,-0.92348601779087));
#55264=DIRECTION('center_axis',(1.,0.,0.));
#55265=DIRECTION('ref_axis',(0.,0.,-1.));
#55266=DIRECTION('center_axis',(-1.,0.,0.));
#55267=DIRECTION('ref_axis',(0.,0.383632082788654,-0.92348601779087));
#55268=DIRECTION('',(0.,0.239315664287559,0.970941817426052));
#55269=DIRECTION('center_axis',(-1.,0.,0.));
#55270=DIRECTION('ref_axis',(0.,0.593489101493642,-0.804842025746835));
#55271=DIRECTION('center_axis',(1.,0.,0.));
#55272=DIRECTION('ref_axis',(0.,0.,-1.));
#55273=DIRECTION('center_axis',(-1.,0.,0.));
#55274=DIRECTION('ref_axis',(0.,0.593489101493642,-0.804842025746835));
#55275=DIRECTION('',(0.,0.,1.));
#55276=DIRECTION('center_axis',(-1.,0.,0.));
#55277=DIRECTION('ref_axis',(0.,1.,0.));
#55278=DIRECTION('center_axis',(1.,0.,0.));
#55279=DIRECTION('ref_axis',(0.,0.995169105836363,0.0981756119861415));
#55280=DIRECTION('center_axis',(1.,0.,0.));
#55281=DIRECTION('ref_axis',(0.,0.995169105836363,0.0981756119861415));
#55282=DIRECTION('',(-1.,0.,0.));
#55283=DIRECTION('center_axis',(-1.,0.,0.));
#55284=DIRECTION('ref_axis',(0.,0.,1.));
#55285=DIRECTION('center_axis',(1.,0.,0.));
#55286=DIRECTION('ref_axis',(0.,0.89953724027626,-0.436844083576932));
#55287=DIRECTION('center_axis',(-1.,0.,0.));
#55288=DIRECTION('ref_axis',(0.,0.89953724027626,-0.436844083576932));
#55289=DIRECTION('',(1.,0.,0.));
#55290=DIRECTION('',(1.,0.,0.));
#55291=DIRECTION('center_axis',(-1.,0.,0.));
#55292=DIRECTION('ref_axis',(0.,0.89953724027626,-0.436844083576932));
#55293=DIRECTION('',(1.,0.,0.));
#55294=DIRECTION('center_axis',(1.,0.,0.));
#55295=DIRECTION('ref_axis',(0.,0.89953724027626,-0.436844083576932));
#55296=DIRECTION('',(-1.,0.,0.));
#55297=DIRECTION('center_axis',(1.,0.,0.));
#55298=DIRECTION('ref_axis',(0.,1.,0.));
#55299=DIRECTION('center_axis',(1.,0.,0.));
#55300=DIRECTION('ref_axis',(0.,0.,-1.));
#55301=DIRECTION('center_axis',(1.,0.,0.));
#55302=DIRECTION('ref_axis',(0.,0.,-1.));
#55303=DIRECTION('center_axis',(1.,0.,0.));
#55304=DIRECTION('ref_axis',(0.,0.,-1.));
#55305=DIRECTION('center_axis',(-1.,0.,0.));
#55306=DIRECTION('ref_axis',(0.,1.,0.));
#55307=DIRECTION('center_axis',(-1.,0.,0.));
#55308=DIRECTION('ref_axis',(0.,0.,1.));
#55309=DIRECTION('center_axis',(1.,0.,0.));
#55310=DIRECTION('ref_axis',(0.,0.97794195496755,-0.208876836231895));
#55311=DIRECTION('center_axis',(-1.,0.,0.));
#55312=DIRECTION('ref_axis',(0.,0.97794195496755,-0.208876836231895));
#55313=DIRECTION('',(1.,0.,0.));
#55314=DIRECTION('',(1.,0.,0.));
#55315=DIRECTION('center_axis',(-1.,0.,0.));
#55316=DIRECTION('ref_axis',(0.,0.97794195496755,-0.208876836231895));
#55317=DIRECTION('',(1.,0.,0.));
#55318=DIRECTION('center_axis',(1.,0.,0.));
#55319=DIRECTION('ref_axis',(0.,0.97794195496755,-0.208876836231895));
#55320=DIRECTION('',(-1.,0.,0.));
#55321=DIRECTION('center_axis',(1.,0.,0.));
#55322=DIRECTION('ref_axis',(0.,1.,0.));
#55323=DIRECTION('center_axis',(1.,0.,0.));
#55324=DIRECTION('ref_axis',(0.,0.,-1.));
#55325=DIRECTION('center_axis',(1.,0.,0.));
#55326=DIRECTION('ref_axis',(0.,0.,-1.));
#55327=DIRECTION('center_axis',(1.,0.,0.));
#55328=DIRECTION('ref_axis',(0.,0.,-1.));
#55329=DIRECTION('center_axis',(-1.,0.,0.));
#55330=DIRECTION('ref_axis',(0.,1.,0.));
#55331=DIRECTION('center_axis',(-1.,0.,0.));
#55332=DIRECTION('ref_axis',(0.,0.,1.));
#55333=DIRECTION('center_axis',(1.,0.,0.));
#55334=DIRECTION('ref_axis',(0.,0.999512237910499,0.0312295735985313));
#55335=DIRECTION('center_axis',(-1.,0.,0.));
#55336=DIRECTION('ref_axis',(0.,0.999512237910499,0.0312295735985313));
#55337=DIRECTION('',(1.,0.,0.));
#55338=DIRECTION('',(1.,0.,0.));
#55339=DIRECTION('center_axis',(-1.,0.,0.));
#55340=DIRECTION('ref_axis',(0.,0.999512237910499,0.0312295735985313));
#55341=DIRECTION('',(1.,0.,0.));
#55342=DIRECTION('center_axis',(1.,0.,0.));
#55343=DIRECTION('ref_axis',(0.,0.999512237910499,0.0312295735985313));
#55344=DIRECTION('',(-1.,0.,0.));
#55345=DIRECTION('center_axis',(1.,0.,0.));
#55346=DIRECTION('ref_axis',(0.,1.,0.));
#55347=DIRECTION('center_axis',(1.,0.,0.));
#55348=DIRECTION('ref_axis',(0.,0.,-1.));
#55349=DIRECTION('center_axis',(1.,0.,0.));
#55350=DIRECTION('ref_axis',(0.,0.,-1.));
#55351=DIRECTION('center_axis',(1.,0.,0.));
#55352=DIRECTION('ref_axis',(0.,0.,-1.));
#55353=DIRECTION('center_axis',(-1.,0.,0.));
#55354=DIRECTION('ref_axis',(0.,1.,0.));
#55355=DIRECTION('center_axis',(-1.,0.,0.));
#55356=DIRECTION('ref_axis',(0.,0.,1.));
#55357=DIRECTION('center_axis',(1.,0.,0.));
#55358=DIRECTION('ref_axis',(0.,0.96299450266525,0.269521034126294));
#55359=DIRECTION('center_axis',(-1.,0.,0.));
#55360=DIRECTION('ref_axis',(0.,0.96299450266525,0.269521034126294));
#55361=DIRECTION('',(1.,0.,0.));
#55362=DIRECTION('',(1.,0.,0.));
#55363=DIRECTION('center_axis',(-1.,0.,0.));
#55364=DIRECTION('ref_axis',(0.,0.96299450266525,0.269521034126294));
#55365=DIRECTION('',(1.,0.,0.));
#55366=DIRECTION('center_axis',(1.,0.,0.));
#55367=DIRECTION('ref_axis',(0.,0.96299450266525,0.269521034126294));
#55368=DIRECTION('',(-1.,0.,0.));
#55369=DIRECTION('center_axis',(1.,0.,0.));
#55370=DIRECTION('ref_axis',(0.,1.,0.));
#55371=DIRECTION('center_axis',(1.,0.,0.));
#55372=DIRECTION('ref_axis',(0.,0.,-1.));
#55373=DIRECTION('center_axis',(1.,0.,0.));
#55374=DIRECTION('ref_axis',(0.,0.,-1.));
#55375=DIRECTION('center_axis',(1.,0.,0.));
#55376=DIRECTION('ref_axis',(0.,0.,-1.));
#55377=DIRECTION('center_axis',(-1.,0.,0.));
#55378=DIRECTION('ref_axis',(0.,1.,0.));
#55379=DIRECTION('center_axis',(-1.,0.,0.));
#55380=DIRECTION('ref_axis',(0.,0.,1.));
#55381=DIRECTION('center_axis',(1.,0.,0.));
#55382=DIRECTION('ref_axis',(0.,0.870511027267693,0.492148911819732));
#55383=DIRECTION('center_axis',(-1.,0.,0.));
#55384=DIRECTION('ref_axis',(0.,0.870511027267693,0.492148911819732));
#55385=DIRECTION('',(1.,0.,0.));
#55386=DIRECTION('',(1.,0.,0.));
#55387=DIRECTION('center_axis',(-1.,0.,0.));
#55388=DIRECTION('ref_axis',(0.,0.870511027267693,0.492148911819732));
#55389=DIRECTION('',(1.,0.,0.));
#55390=DIRECTION('center_axis',(1.,0.,0.));
#55391=DIRECTION('ref_axis',(0.,0.870511027267693,0.492148911819732));
#55392=DIRECTION('',(-1.,0.,0.));
#55393=DIRECTION('center_axis',(1.,0.,0.));
#55394=DIRECTION('ref_axis',(0.,1.,0.));
#55395=DIRECTION('center_axis',(1.,0.,0.));
#55396=DIRECTION('ref_axis',(0.,0.,-1.));
#55397=DIRECTION('center_axis',(1.,0.,0.));
#55398=DIRECTION('ref_axis',(0.,0.,-1.));
#55399=DIRECTION('center_axis',(1.,0.,0.));
#55400=DIRECTION('ref_axis',(0.,0.,-1.));
#55401=DIRECTION('center_axis',(-1.,0.,0.));
#55402=DIRECTION('ref_axis',(0.,1.,0.));
#55403=DIRECTION('center_axis',(-1.,0.,0.));
#55404=DIRECTION('ref_axis',(0.,0.,1.));
#55405=DIRECTION('center_axis',(1.,0.,0.));
#55406=DIRECTION('ref_axis',(0.,0.727436615144173,0.686174883646719));
#55407=DIRECTION('center_axis',(-1.,0.,0.));
#55408=DIRECTION('ref_axis',(0.,0.727436615144173,0.686174883646719));
#55409=DIRECTION('',(1.,0.,0.));
#55410=DIRECTION('',(1.,0.,0.));
#55411=DIRECTION('center_axis',(-1.,0.,0.));
#55412=DIRECTION('ref_axis',(0.,0.727436615144173,0.686174883646719));
#55413=DIRECTION('',(1.,0.,0.));
#55414=DIRECTION('center_axis',(1.,0.,0.));
#55415=DIRECTION('ref_axis',(0.,0.727436615144173,0.686174883646719));
#55416=DIRECTION('',(-1.,0.,0.));
#55417=DIRECTION('center_axis',(1.,0.,0.));
#55418=DIRECTION('ref_axis',(0.,1.,0.));
#55419=DIRECTION('center_axis',(1.,0.,0.));
#55420=DIRECTION('ref_axis',(0.,0.,-1.));
#55421=DIRECTION('center_axis',(1.,0.,0.));
#55422=DIRECTION('ref_axis',(0.,0.,-1.));
#55423=DIRECTION('center_axis',(1.,0.,0.));
#55424=DIRECTION('ref_axis',(0.,0.,-1.));
#55425=DIRECTION('center_axis',(-1.,0.,0.));
#55426=DIRECTION('ref_axis',(0.,1.,0.));
#55427=DIRECTION('center_axis',(-1.,0.,0.));
#55428=DIRECTION('ref_axis',(0.,0.,1.));
#55429=DIRECTION('center_axis',(1.,0.,0.));
#55430=DIRECTION('ref_axis',(0.,0.542086231072989,0.840322865380374));
#55431=DIRECTION('center_axis',(-1.,0.,0.));
#55432=DIRECTION('ref_axis',(0.,0.542086231072989,0.840322865380374));
#55433=DIRECTION('',(1.,0.,0.));
#55434=DIRECTION('',(1.,0.,0.));
#55435=DIRECTION('center_axis',(-1.,0.,0.));
#55436=DIRECTION('ref_axis',(0.,0.542086231072989,0.840322865380374));
#55437=DIRECTION('',(1.,0.,0.));
#55438=DIRECTION('center_axis',(1.,0.,0.));
#55439=DIRECTION('ref_axis',(0.,0.542086231072989,0.840322865380374));
#55440=DIRECTION('',(-1.,0.,0.));
#55441=DIRECTION('center_axis',(1.,0.,0.));
#55442=DIRECTION('ref_axis',(0.,1.,0.));
#55443=DIRECTION('center_axis',(1.,0.,0.));
#55444=DIRECTION('ref_axis',(0.,0.,-1.));
#55445=DIRECTION('center_axis',(1.,0.,0.));
#55446=DIRECTION('ref_axis',(0.,0.,-1.));
#55447=DIRECTION('center_axis',(1.,0.,0.));
#55448=DIRECTION('ref_axis',(0.,0.,-1.));
#55449=DIRECTION('center_axis',(-1.,0.,0.));
#55450=DIRECTION('ref_axis',(0.,1.,0.));
#55451=DIRECTION('center_axis',(-1.,0.,0.));
#55452=DIRECTION('ref_axis',(0.,0.,1.));
#55453=DIRECTION('center_axis',(1.,0.,0.));
#55454=DIRECTION('ref_axis',(0.,0.325231765655118,0.945634336627459));
#55455=DIRECTION('center_axis',(-1.,0.,0.));
#55456=DIRECTION('ref_axis',(0.,0.325231765655118,0.945634336627459));
#55457=DIRECTION('',(1.,0.,0.));
#55458=DIRECTION('',(1.,0.,0.));
#55459=DIRECTION('center_axis',(-1.,0.,0.));
#55460=DIRECTION('ref_axis',(0.,0.325231765655118,0.945634336627459));
#55461=DIRECTION('',(1.,0.,0.));
#55462=DIRECTION('center_axis',(1.,0.,0.));
#55463=DIRECTION('ref_axis',(0.,0.325231765655118,0.945634336627459));
#55464=DIRECTION('',(-1.,0.,0.));
#55465=DIRECTION('center_axis',(1.,0.,0.));
#55466=DIRECTION('ref_axis',(0.,1.,0.));
#55467=DIRECTION('center_axis',(1.,0.,0.));
#55468=DIRECTION('ref_axis',(0.,0.,-1.));
#55469=DIRECTION('center_axis',(1.,0.,0.));
#55470=DIRECTION('ref_axis',(0.,0.,-1.));
#55471=DIRECTION('center_axis',(1.,0.,0.));
#55472=DIRECTION('ref_axis',(0.,0.,-1.));
#55473=DIRECTION('center_axis',(-1.,0.,0.));
#55474=DIRECTION('ref_axis',(0.,1.,0.));
#55475=DIRECTION('center_axis',(-1.,0.,0.));
#55476=DIRECTION('ref_axis',(0.,0.,1.));
#55477=DIRECTION('center_axis',(1.,0.,0.));
#55478=DIRECTION('ref_axis',(0.,0.0894760121867377,0.995988977470714));
#55479=DIRECTION('center_axis',(-1.,0.,0.));
#55480=DIRECTION('ref_axis',(0.,0.0894760121867377,0.995988977470714));
#55481=DIRECTION('',(1.,0.,0.));
#55482=DIRECTION('',(1.,0.,0.));
#55483=DIRECTION('center_axis',(-1.,0.,0.));
#55484=DIRECTION('ref_axis',(0.,0.0894760121867377,0.995988977470714));
#55485=DIRECTION('',(1.,0.,0.));
#55486=DIRECTION('center_axis',(1.,0.,0.));
#55487=DIRECTION('ref_axis',(0.,0.0894760121867377,0.995988977470714));
#55488=DIRECTION('',(-1.,0.,0.));
#55489=DIRECTION('center_axis',(1.,0.,0.));
#55490=DIRECTION('ref_axis',(0.,1.,0.));
#55491=DIRECTION('center_axis',(1.,0.,0.));
#55492=DIRECTION('ref_axis',(0.,0.,-1.));
#55493=DIRECTION('center_axis',(1.,0.,0.));
#55494=DIRECTION('ref_axis',(0.,0.,-1.));
#55495=DIRECTION('center_axis',(1.,0.,0.));
#55496=DIRECTION('ref_axis',(0.,0.,-1.));
#55497=DIRECTION('center_axis',(-1.,0.,0.));
#55498=DIRECTION('ref_axis',(0.,1.,0.));
#55499=DIRECTION('center_axis',(-1.,0.,0.));
#55500=DIRECTION('ref_axis',(0.,0.,1.));
#55501=DIRECTION('center_axis',(1.,0.,0.));
#55502=DIRECTION('ref_axis',(0.,-0.151479761877859,0.988460359216002));
#55503=DIRECTION('center_axis',(-1.,0.,0.));
#55504=DIRECTION('ref_axis',(0.,-0.151479761877859,0.988460359216002));
#55505=DIRECTION('',(1.,0.,0.));
#55506=DIRECTION('',(1.,0.,0.));
#55507=DIRECTION('center_axis',(-1.,0.,0.));
#55508=DIRECTION('ref_axis',(0.,-0.151479761877859,0.988460359216002));
#55509=DIRECTION('',(1.,0.,0.));
#55510=DIRECTION('center_axis',(1.,0.,0.));
#55511=DIRECTION('ref_axis',(0.,-0.151479761877859,0.988460359216002));
#55512=DIRECTION('',(-1.,0.,0.));
#55513=DIRECTION('center_axis',(1.,0.,0.));
#55514=DIRECTION('ref_axis',(0.,1.,0.));
#55515=DIRECTION('center_axis',(1.,0.,0.));
#55516=DIRECTION('ref_axis',(0.,0.,-1.));
#55517=DIRECTION('center_axis',(1.,0.,0.));
#55518=DIRECTION('ref_axis',(0.,0.,-1.));
#55519=DIRECTION('center_axis',(1.,0.,0.));
#55520=DIRECTION('ref_axis',(0.,0.,-1.));
#55521=DIRECTION('center_axis',(-1.,0.,0.));
#55522=DIRECTION('ref_axis',(0.,1.,0.));
#55523=DIRECTION('center_axis',(-1.,0.,0.));
#55524=DIRECTION('ref_axis',(0.,0.,1.));
#55525=DIRECTION('center_axis',(1.,0.,0.));
#55526=DIRECTION('ref_axis',(0.,-0.383632082788652,0.923486017790871));
#55527=DIRECTION('center_axis',(-1.,0.,0.));
#55528=DIRECTION('ref_axis',(0.,-0.383632082788652,0.923486017790871));
#55529=DIRECTION('',(1.,0.,0.));
#55530=DIRECTION('',(1.,0.,0.));
#55531=DIRECTION('center_axis',(-1.,0.,0.));
#55532=DIRECTION('ref_axis',(0.,-0.383632082788652,0.923486017790871));
#55533=DIRECTION('',(1.,0.,0.));
#55534=DIRECTION('center_axis',(1.,0.,0.));
#55535=DIRECTION('ref_axis',(0.,-0.383632082788652,0.923486017790871));
#55536=DIRECTION('',(-1.,0.,0.));
#55537=DIRECTION('center_axis',(1.,0.,0.));
#55538=DIRECTION('ref_axis',(0.,1.,0.));
#55539=DIRECTION('center_axis',(1.,0.,0.));
#55540=DIRECTION('ref_axis',(0.,0.,-1.));
#55541=DIRECTION('center_axis',(1.,0.,0.));
#55542=DIRECTION('ref_axis',(0.,0.,-1.));
#55543=DIRECTION('center_axis',(1.,0.,0.));
#55544=DIRECTION('ref_axis',(0.,0.,-1.));
#55545=DIRECTION('center_axis',(-1.,0.,0.));
#55546=DIRECTION('ref_axis',(0.,1.,0.));
#55547=DIRECTION('center_axis',(-1.,0.,0.));
#55548=DIRECTION('ref_axis',(0.,0.,1.));
#55549=DIRECTION('center_axis',(1.,0.,0.));
#55550=DIRECTION('ref_axis',(0.,-0.593489101493646,0.804842025746833));
#55551=DIRECTION('center_axis',(-1.,0.,0.));
#55552=DIRECTION('ref_axis',(0.,-0.593489101493646,0.804842025746833));
#55553=DIRECTION('',(1.,0.,0.));
#55554=DIRECTION('',(1.,0.,0.));
#55555=DIRECTION('center_axis',(-1.,0.,0.));
#55556=DIRECTION('ref_axis',(0.,-0.593489101493646,0.804842025746833));
#55557=DIRECTION('',(1.,0.,0.));
#55558=DIRECTION('center_axis',(1.,0.,0.));
#55559=DIRECTION('ref_axis',(0.,-0.593489101493646,0.804842025746833));
#55560=DIRECTION('',(-1.,0.,0.));
#55561=DIRECTION('center_axis',(1.,0.,0.));
#55562=DIRECTION('ref_axis',(0.,1.,0.));
#55563=DIRECTION('center_axis',(1.,0.,0.));
#55564=DIRECTION('ref_axis',(0.,0.,-1.));
#55565=DIRECTION('center_axis',(1.,0.,0.));
#55566=DIRECTION('ref_axis',(0.,0.,-1.));
#55567=DIRECTION('center_axis',(1.,0.,0.));
#55568=DIRECTION('ref_axis',(0.,0.,-1.));
#55569=DIRECTION('center_axis',(-1.,0.,0.));
#55570=DIRECTION('ref_axis',(0.,1.,0.));
#55571=DIRECTION('center_axis',(-1.,0.,0.));
#55572=DIRECTION('ref_axis',(0.,0.,1.));
#55573=DIRECTION('center_axis',(1.,0.,0.));
#55574=DIRECTION('ref_axis',(0.,-0.768854690864945,0.639423540648114));
#55575=DIRECTION('center_axis',(-1.,0.,0.));
#55576=DIRECTION('ref_axis',(0.,-0.768854690864945,0.639423540648114));
#55577=DIRECTION('',(1.,0.,0.));
#55578=DIRECTION('',(1.,0.,0.));
#55579=DIRECTION('center_axis',(-1.,0.,0.));
#55580=DIRECTION('ref_axis',(0.,-0.768854690864945,0.639423540648114));
#55581=DIRECTION('',(1.,0.,0.));
#55582=DIRECTION('center_axis',(1.,0.,0.));
#55583=DIRECTION('ref_axis',(0.,-0.768854690864945,0.639423540648114));
#55584=DIRECTION('',(-1.,0.,0.));
#55585=DIRECTION('center_axis',(1.,0.,0.));
#55586=DIRECTION('ref_axis',(0.,1.,0.));
#55587=DIRECTION('center_axis',(1.,0.,0.));
#55588=DIRECTION('ref_axis',(0.,0.,-1.));
#55589=DIRECTION('center_axis',(1.,0.,0.));
#55590=DIRECTION('ref_axis',(0.,0.,-1.));
#55591=DIRECTION('center_axis',(1.,0.,0.));
#55592=DIRECTION('ref_axis',(0.,0.,-1.));
#55593=DIRECTION('center_axis',(-1.,0.,0.));
#55594=DIRECTION('ref_axis',(0.,1.,0.));
#55595=DIRECTION('center_axis',(-1.,0.,0.));
#55596=DIRECTION('ref_axis',(0.,0.,1.));
#55597=DIRECTION('center_axis',(1.,0.,0.));
#55598=DIRECTION('ref_axis',(0.,-0.899537240276258,0.436844083576936));
#55599=DIRECTION('center_axis',(-1.,0.,0.));
#55600=DIRECTION('ref_axis',(0.,-0.899537240276258,0.436844083576936));
#55601=DIRECTION('',(1.,0.,0.));
#55602=DIRECTION('',(1.,0.,0.));
#55603=DIRECTION('center_axis',(-1.,0.,0.));
#55604=DIRECTION('ref_axis',(0.,-0.899537240276258,0.436844083576936));
#55605=DIRECTION('',(1.,0.,0.));
#55606=DIRECTION('center_axis',(1.,0.,0.));
#55607=DIRECTION('ref_axis',(0.,-0.899537240276258,0.436844083576936));
#55608=DIRECTION('',(-1.,0.,0.));
#55609=DIRECTION('center_axis',(1.,0.,0.));
#55610=DIRECTION('ref_axis',(0.,1.,0.));
#55611=DIRECTION('center_axis',(1.,0.,0.));
#55612=DIRECTION('ref_axis',(0.,0.,-1.));
#55613=DIRECTION('center_axis',(1.,0.,0.));
#55614=DIRECTION('ref_axis',(0.,0.,-1.));
#55615=DIRECTION('center_axis',(1.,0.,0.));
#55616=DIRECTION('ref_axis',(0.,0.,-1.));
#55617=DIRECTION('center_axis',(-1.,0.,0.));
#55618=DIRECTION('ref_axis',(0.,1.,0.));
#55619=DIRECTION('center_axis',(-1.,0.,0.));
#55620=DIRECTION('ref_axis',(0.,0.,1.));
#55621=DIRECTION('center_axis',(1.,0.,0.));
#55622=DIRECTION('ref_axis',(0.,-0.97794195496755,0.208876836231895));
#55623=DIRECTION('center_axis',(-1.,0.,0.));
#55624=DIRECTION('ref_axis',(0.,-0.97794195496755,0.208876836231895));
#55625=DIRECTION('',(1.,0.,0.));
#55626=DIRECTION('',(1.,0.,0.));
#55627=DIRECTION('center_axis',(-1.,0.,0.));
#55628=DIRECTION('ref_axis',(0.,-0.97794195496755,0.208876836231895));
#55629=DIRECTION('',(1.,0.,0.));
#55630=DIRECTION('center_axis',(1.,0.,0.));
#55631=DIRECTION('ref_axis',(0.,-0.97794195496755,0.208876836231895));
#55632=DIRECTION('',(-1.,0.,0.));
#55633=DIRECTION('center_axis',(1.,0.,0.));
#55634=DIRECTION('ref_axis',(0.,1.,0.));
#55635=DIRECTION('center_axis',(1.,0.,0.));
#55636=DIRECTION('ref_axis',(0.,0.,-1.));
#55637=DIRECTION('center_axis',(1.,0.,0.));
#55638=DIRECTION('ref_axis',(0.,0.,-1.));
#55639=DIRECTION('center_axis',(1.,0.,0.));
#55640=DIRECTION('ref_axis',(0.,0.,-1.));
#55641=DIRECTION('center_axis',(-1.,0.,0.));
#55642=DIRECTION('ref_axis',(0.,1.,0.));
#55643=DIRECTION('center_axis',(-1.,0.,0.));
#55644=DIRECTION('ref_axis',(0.,0.,1.));
#55645=DIRECTION('center_axis',(1.,0.,0.));
#55646=DIRECTION('ref_axis',(0.,-0.999512237910499,-0.0312295735985302));
#55647=DIRECTION('center_axis',(-1.,0.,0.));
#55648=DIRECTION('ref_axis',(0.,-0.999512237910499,-0.0312295735985302));
#55649=DIRECTION('',(1.,0.,0.));
#55650=DIRECTION('',(1.,0.,0.));
#55651=DIRECTION('center_axis',(-1.,0.,0.));
#55652=DIRECTION('ref_axis',(0.,-0.999512237910499,-0.0312295735985302));
#55653=DIRECTION('',(1.,0.,0.));
#55654=DIRECTION('center_axis',(1.,0.,0.));
#55655=DIRECTION('ref_axis',(0.,-0.999512237910499,-0.0312295735985302));
#55656=DIRECTION('',(-1.,0.,0.));
#55657=DIRECTION('center_axis',(1.,0.,0.));
#55658=DIRECTION('ref_axis',(0.,1.,0.));
#55659=DIRECTION('center_axis',(1.,0.,0.));
#55660=DIRECTION('ref_axis',(0.,0.,-1.));
#55661=DIRECTION('center_axis',(1.,0.,0.));
#55662=DIRECTION('ref_axis',(0.,0.,-1.));
#55663=DIRECTION('center_axis',(1.,0.,0.));
#55664=DIRECTION('ref_axis',(0.,0.,-1.));
#55665=DIRECTION('center_axis',(-1.,0.,0.));
#55666=DIRECTION('ref_axis',(0.,1.,0.));
#55667=DIRECTION('center_axis',(-1.,0.,0.));
#55668=DIRECTION('ref_axis',(0.,0.,1.));
#55669=DIRECTION('center_axis',(1.,0.,0.));
#55670=DIRECTION('ref_axis',(0.,-0.96299450266525,-0.269521034126296));
#55671=DIRECTION('center_axis',(-1.,0.,0.));
#55672=DIRECTION('ref_axis',(0.,-0.96299450266525,-0.269521034126296));
#55673=DIRECTION('',(1.,0.,0.));
#55674=DIRECTION('',(1.,0.,0.));
#55675=DIRECTION('center_axis',(-1.,0.,0.));
#55676=DIRECTION('ref_axis',(0.,-0.96299450266525,-0.269521034126296));
#55677=DIRECTION('',(1.,0.,0.));
#55678=DIRECTION('center_axis',(1.,0.,0.));
#55679=DIRECTION('ref_axis',(0.,-0.96299450266525,-0.269521034126296));
#55680=DIRECTION('',(-1.,0.,0.));
#55681=DIRECTION('center_axis',(1.,0.,0.));
#55682=DIRECTION('ref_axis',(0.,1.,0.));
#55683=DIRECTION('center_axis',(1.,0.,0.));
#55684=DIRECTION('ref_axis',(0.,0.,-1.));
#55685=DIRECTION('center_axis',(1.,0.,0.));
#55686=DIRECTION('ref_axis',(0.,0.,-1.));
#55687=DIRECTION('center_axis',(1.,0.,0.));
#55688=DIRECTION('ref_axis',(0.,0.,-1.));
#55689=DIRECTION('center_axis',(-1.,0.,0.));
#55690=DIRECTION('ref_axis',(0.,1.,0.));
#55691=DIRECTION('center_axis',(-1.,0.,0.));
#55692=DIRECTION('ref_axis',(0.,0.,1.));
#55693=DIRECTION('center_axis',(1.,0.,0.));
#55694=DIRECTION('ref_axis',(0.,-0.87051102726769,-0.492148911819736));
#55695=DIRECTION('center_axis',(-1.,0.,0.));
#55696=DIRECTION('ref_axis',(0.,-0.87051102726769,-0.492148911819736));
#55697=DIRECTION('',(1.,0.,0.));
#55698=DIRECTION('',(1.,0.,0.));
#55699=DIRECTION('center_axis',(-1.,0.,0.));
#55700=DIRECTION('ref_axis',(0.,-0.87051102726769,-0.492148911819736));
#55701=DIRECTION('',(1.,0.,0.));
#55702=DIRECTION('center_axis',(1.,0.,0.));
#55703=DIRECTION('ref_axis',(0.,-0.87051102726769,-0.492148911819736));
#55704=DIRECTION('',(-1.,0.,0.));
#55705=DIRECTION('center_axis',(1.,0.,0.));
#55706=DIRECTION('ref_axis',(0.,1.,0.));
#55707=DIRECTION('center_axis',(1.,0.,0.));
#55708=DIRECTION('ref_axis',(0.,0.,-1.));
#55709=DIRECTION('center_axis',(1.,0.,0.));
#55710=DIRECTION('ref_axis',(0.,0.,-1.));
#55711=DIRECTION('center_axis',(1.,0.,0.));
#55712=DIRECTION('ref_axis',(0.,0.,-1.));
#55713=DIRECTION('center_axis',(-1.,0.,0.));
#55714=DIRECTION('ref_axis',(0.,1.,0.));
#55715=DIRECTION('center_axis',(-1.,0.,0.));
#55716=DIRECTION('ref_axis',(0.,0.,1.));
#55717=DIRECTION('center_axis',(1.,0.,0.));
#55718=DIRECTION('ref_axis',(0.,-0.727436615144171,-0.686174883646721));
#55719=DIRECTION('center_axis',(-1.,0.,0.));
#55720=DIRECTION('ref_axis',(0.,-0.727436615144171,-0.686174883646721));
#55721=DIRECTION('',(1.,0.,0.));
#55722=DIRECTION('',(1.,0.,0.));
#55723=DIRECTION('center_axis',(-1.,0.,0.));
#55724=DIRECTION('ref_axis',(0.,-0.727436615144171,-0.686174883646721));
#55725=DIRECTION('',(1.,0.,0.));
#55726=DIRECTION('center_axis',(1.,0.,0.));
#55727=DIRECTION('ref_axis',(0.,-0.727436615144171,-0.686174883646721));
#55728=DIRECTION('',(-1.,0.,0.));
#55729=DIRECTION('center_axis',(1.,0.,0.));
#55730=DIRECTION('ref_axis',(0.,1.,0.));
#55731=DIRECTION('center_axis',(1.,0.,0.));
#55732=DIRECTION('ref_axis',(0.,0.,-1.));
#55733=DIRECTION('center_axis',(1.,0.,0.));
#55734=DIRECTION('ref_axis',(0.,0.,-1.));
#55735=DIRECTION('center_axis',(1.,0.,0.));
#55736=DIRECTION('ref_axis',(0.,0.,-1.));
#55737=DIRECTION('center_axis',(-1.,0.,0.));
#55738=DIRECTION('ref_axis',(0.,1.,0.));
#55739=DIRECTION('center_axis',(-1.,0.,0.));
#55740=DIRECTION('ref_axis',(0.,0.,1.));
#55741=DIRECTION('center_axis',(1.,0.,0.));
#55742=DIRECTION('ref_axis',(0.,-0.542086231072992,-0.840322865380372));
#55743=DIRECTION('center_axis',(-1.,0.,0.));
#55744=DIRECTION('ref_axis',(0.,-0.542086231072992,-0.840322865380372));
#55745=DIRECTION('',(1.,0.,0.));
#55746=DIRECTION('',(1.,0.,0.));
#55747=DIRECTION('center_axis',(-1.,0.,0.));
#55748=DIRECTION('ref_axis',(0.,-0.542086231072992,-0.840322865380372));
#55749=DIRECTION('',(1.,0.,0.));
#55750=DIRECTION('center_axis',(1.,0.,0.));
#55751=DIRECTION('ref_axis',(0.,-0.542086231072992,-0.840322865380372));
#55752=DIRECTION('',(-1.,0.,0.));
#55753=DIRECTION('center_axis',(1.,0.,0.));
#55754=DIRECTION('ref_axis',(0.,1.,0.));
#55755=DIRECTION('center_axis',(1.,0.,0.));
#55756=DIRECTION('ref_axis',(0.,0.,-1.));
#55757=DIRECTION('center_axis',(1.,0.,0.));
#55758=DIRECTION('ref_axis',(0.,0.,-1.));
#55759=DIRECTION('center_axis',(1.,0.,0.));
#55760=DIRECTION('ref_axis',(0.,0.,-1.));
#55761=DIRECTION('center_axis',(-1.,0.,0.));
#55762=DIRECTION('ref_axis',(0.,1.,0.));
#55763=DIRECTION('center_axis',(-1.,0.,0.));
#55764=DIRECTION('ref_axis',(0.,0.,1.));
#55765=DIRECTION('center_axis',(1.,0.,0.));
#55766=DIRECTION('ref_axis',(0.,-0.325231765655117,-0.945634336627459));
#55767=DIRECTION('center_axis',(-1.,0.,0.));
#55768=DIRECTION('ref_axis',(0.,-0.325231765655117,-0.945634336627459));
#55769=DIRECTION('',(1.,0.,0.));
#55770=DIRECTION('',(1.,0.,0.));
#55771=DIRECTION('center_axis',(-1.,0.,0.));
#55772=DIRECTION('ref_axis',(0.,-0.325231765655117,-0.945634336627459));
#55773=DIRECTION('',(1.,0.,0.));
#55774=DIRECTION('center_axis',(1.,0.,0.));
#55775=DIRECTION('ref_axis',(0.,-0.325231765655117,-0.945634336627459));
#55776=DIRECTION('',(-1.,0.,0.));
#55777=DIRECTION('center_axis',(1.,0.,0.));
#55778=DIRECTION('ref_axis',(0.,1.,0.));
#55779=DIRECTION('center_axis',(1.,0.,0.));
#55780=DIRECTION('ref_axis',(0.,0.,-1.));
#55781=DIRECTION('center_axis',(1.,0.,0.));
#55782=DIRECTION('ref_axis',(0.,0.,-1.));
#55783=DIRECTION('center_axis',(1.,0.,0.));
#55784=DIRECTION('ref_axis',(0.,0.,-1.));
#55785=DIRECTION('center_axis',(-1.,0.,0.));
#55786=DIRECTION('ref_axis',(0.,1.,0.));
#55787=DIRECTION('center_axis',(-1.,0.,0.));
#55788=DIRECTION('ref_axis',(0.,0.,1.));
#55789=DIRECTION('center_axis',(1.,0.,0.));
#55790=DIRECTION('ref_axis',(0.,-0.0894760121867388,-0.995988977470714));
#55791=DIRECTION('center_axis',(-1.,0.,0.));
#55792=DIRECTION('ref_axis',(0.,-0.0894760121867388,-0.995988977470714));
#55793=DIRECTION('',(1.,0.,0.));
#55794=DIRECTION('',(1.,0.,0.));
#55795=DIRECTION('center_axis',(-1.,0.,0.));
#55796=DIRECTION('ref_axis',(0.,-0.0894760121867388,-0.995988977470714));
#55797=DIRECTION('',(1.,0.,0.));
#55798=DIRECTION('center_axis',(1.,0.,0.));
#55799=DIRECTION('ref_axis',(0.,-0.0894760121867388,-0.995988977470714));
#55800=DIRECTION('',(-1.,0.,0.));
#55801=DIRECTION('center_axis',(1.,0.,0.));
#55802=DIRECTION('ref_axis',(0.,1.,0.));
#55803=DIRECTION('center_axis',(1.,0.,0.));
#55804=DIRECTION('ref_axis',(0.,0.,-1.));
#55805=DIRECTION('center_axis',(1.,0.,0.));
#55806=DIRECTION('ref_axis',(0.,0.,-1.));
#55807=DIRECTION('center_axis',(1.,0.,0.));
#55808=DIRECTION('ref_axis',(0.,0.,-1.));
#55809=DIRECTION('center_axis',(-1.,0.,0.));
#55810=DIRECTION('ref_axis',(0.,1.,0.));
#55811=DIRECTION('center_axis',(-1.,0.,0.));
#55812=DIRECTION('ref_axis',(0.,0.,1.));
#55813=DIRECTION('center_axis',(1.,0.,0.));
#55814=DIRECTION('ref_axis',(0.,0.151479761877861,-0.988460359216002));
#55815=DIRECTION('center_axis',(-1.,0.,0.));
#55816=DIRECTION('ref_axis',(0.,0.151479761877861,-0.988460359216002));
#55817=DIRECTION('',(1.,0.,0.));
#55818=DIRECTION('',(1.,0.,0.));
#55819=DIRECTION('center_axis',(-1.,0.,0.));
#55820=DIRECTION('ref_axis',(0.,0.151479761877861,-0.988460359216002));
#55821=DIRECTION('',(1.,0.,0.));
#55822=DIRECTION('center_axis',(1.,0.,0.));
#55823=DIRECTION('ref_axis',(0.,0.151479761877861,-0.988460359216002));
#55824=DIRECTION('',(-1.,0.,0.));
#55825=DIRECTION('center_axis',(1.,0.,0.));
#55826=DIRECTION('ref_axis',(0.,1.,0.));
#55827=DIRECTION('center_axis',(1.,0.,0.));
#55828=DIRECTION('ref_axis',(0.,0.,-1.));
#55829=DIRECTION('center_axis',(1.,0.,0.));
#55830=DIRECTION('ref_axis',(0.,0.,-1.));
#55831=DIRECTION('center_axis',(1.,0.,0.));
#55832=DIRECTION('ref_axis',(0.,0.,-1.));
#55833=DIRECTION('center_axis',(-1.,0.,0.));
#55834=DIRECTION('ref_axis',(0.,1.,0.));
#55835=DIRECTION('center_axis',(-1.,0.,0.));
#55836=DIRECTION('ref_axis',(0.,0.,1.));
#55837=DIRECTION('center_axis',(1.,0.,0.));
#55838=DIRECTION('ref_axis',(0.,0.593489101493642,-0.804842025746835));
#55839=DIRECTION('center_axis',(-1.,0.,0.));
#55840=DIRECTION('ref_axis',(0.,0.593489101493642,-0.804842025746835));
#55841=DIRECTION('',(1.,0.,0.));
#55842=DIRECTION('',(1.,0.,0.));
#55843=DIRECTION('center_axis',(-1.,0.,0.));
#55844=DIRECTION('ref_axis',(0.,0.593489101493642,-0.804842025746835));
#55845=DIRECTION('',(1.,0.,0.));
#55846=DIRECTION('center_axis',(1.,0.,0.));
#55847=DIRECTION('ref_axis',(0.,0.593489101493642,-0.804842025746835));
#55848=DIRECTION('',(-1.,0.,0.));
#55849=DIRECTION('center_axis',(-1.,0.,0.));
#55850=DIRECTION('ref_axis',(0.,1.,0.));
#55851=DIRECTION('center_axis',(1.,0.,0.));
#55852=DIRECTION('ref_axis',(0.,1.,0.));
#55853=DIRECTION('center_axis',(1.,0.,0.));
#55854=DIRECTION('ref_axis',(0.,0.,-1.));
#55855=DIRECTION('center_axis',(1.,0.,0.));
#55856=DIRECTION('ref_axis',(0.,0.,-1.));
#55857=DIRECTION('center_axis',(1.,0.,0.));
#55858=DIRECTION('ref_axis',(0.,0.,-1.));
#55859=DIRECTION('center_axis',(1.,0.,0.));
#55860=DIRECTION('ref_axis',(0.,0.383632082788654,-0.92348601779087));
#55861=DIRECTION('center_axis',(-1.,0.,0.));
#55862=DIRECTION('ref_axis',(0.,0.383632082788654,-0.92348601779087));
#55863=DIRECTION('',(1.,0.,0.));
#55864=DIRECTION('',(1.,0.,0.));
#55865=DIRECTION('center_axis',(-1.,0.,0.));
#55866=DIRECTION('ref_axis',(0.,0.383632082788654,-0.92348601779087));
#55867=DIRECTION('',(1.,0.,0.));
#55868=DIRECTION('center_axis',(1.,0.,0.));
#55869=DIRECTION('ref_axis',(0.,0.383632082788654,-0.92348601779087));
#55870=DIRECTION('',(-1.,0.,0.));
#55871=DIRECTION('center_axis',(1.,0.,0.));
#55872=DIRECTION('ref_axis',(0.,1.,0.));
#55873=DIRECTION('center_axis',(1.,0.,0.));
#55874=DIRECTION('ref_axis',(0.,0.,-1.));
#55875=DIRECTION('center_axis',(1.,0.,0.));
#55876=DIRECTION('ref_axis',(0.,0.,-1.));
#55877=DIRECTION('center_axis',(1.,0.,0.));
#55878=DIRECTION('ref_axis',(0.,0.,-1.));
#55879=DIRECTION('center_axis',(1.,0.,0.));
#55880=DIRECTION('ref_axis',(0.,0.,-1.));
#55881=DIRECTION('center_axis',(-1.,0.,0.));
#55882=DIRECTION('ref_axis',(0.,-1.,1.83697019872103E-16));
#55883=DIRECTION('center_axis',(0.,-1.,-1.22464679914735E-16));
#55884=DIRECTION('ref_axis',(0.,-1.22464679914735E-16,1.));
#55885=DIRECTION('center_axis',(1.,0.,0.));
#55886=DIRECTION('ref_axis',(0.,-1.,1.83697019872103E-16));
#55887=DIRECTION('center_axis',(1.,0.,0.));
#55888=DIRECTION('ref_axis',(0.,-1.,1.83697019872103E-16));
#55889=DIRECTION('center_axis',(-1.,0.,0.));
#55890=DIRECTION('ref_axis',(0.,-1.,1.83697019872103E-16));
#55891=DIRECTION('center_axis',(1.,0.,0.));
#55892=DIRECTION('ref_axis',(0.,1.,0.));
#55893=DIRECTION('center_axis',(1.,0.,0.));
#55894=DIRECTION('ref_axis',(0.,0.,-1.));
#55895=DIRECTION('center_axis',(1.,0.,0.));
#55896=DIRECTION('ref_axis',(0.,1.,0.));
#55897=DIRECTION('',(0.,0.,-1.));
#55898=DIRECTION('',(0.,-0.239315664287559,-0.970941817426052));
#55899=DIRECTION('',(0.,-0.464723172043769,-0.88545602565321));
#55900=DIRECTION('',(0.,-0.663122658240796,-0.748510748171101));
#55901=DIRECTION('',(0.,-0.822983865893656,-0.568064746731156));
#55902=DIRECTION('',(0.,-0.935016242685415,-0.354604887042536));
#55903=DIRECTION('',(0.,-0.992708874098054,-0.120536680255322));
#55904=DIRECTION('',(0.,-0.992708874098054,0.120536680255324));
#55905=DIRECTION('',(0.,-0.935016242685415,0.354604887042536));
#55906=DIRECTION('',(0.,-0.822983865893656,0.568064746731156));
#55907=DIRECTION('',(0.,-0.663122658240795,0.748510748171101));
#55908=DIRECTION('',(0.,-0.464723172043768,0.88545602565321));
#55909=DIRECTION('',(0.,-0.239315664287557,0.970941817426052));
#55910=DIRECTION('',(0.,1.22464679914735E-16,1.));
#55911=DIRECTION('',(0.,0.239315664287558,0.970941817426052));
#55912=DIRECTION('',(0.,0.464723172043769,0.88545602565321));
#55913=DIRECTION('',(0.,0.663122658240796,0.748510748171101));
#55914=DIRECTION('',(0.,0.822983865893656,0.568064746731156));
#55915=DIRECTION('',(0.,0.935016242685415,0.354604887042536));
#55916=DIRECTION('',(0.,0.992708874098054,0.120536680255323));
#55917=DIRECTION('',(0.,0.992708874098054,-0.120536680255323));
#55918=DIRECTION('',(0.,0.935016242685415,-0.354604887042536));
#55919=DIRECTION('',(0.,0.822983865893656,-0.568064746731156));
#55920=DIRECTION('',(0.,0.663122658240795,-0.748510748171101));
#55921=DIRECTION('',(0.,0.464723172043769,-0.88545602565321));
#55922=DIRECTION('',(0.,0.239315664287558,-0.970941817426052));
#55923=DIRECTION('center_axis',(1.,0.,0.));
#55924=DIRECTION('ref_axis',(0.,1.,0.));
#55925=DIRECTION('',(-1.,0.,0.));
#55926=DIRECTION('center_axis',(-1.,0.,0.));
#55927=DIRECTION('ref_axis',(0.,1.,0.));
#55928=DIRECTION('center_axis',(0.,-0.970941817426052,0.239315664287559));
#55929=DIRECTION('ref_axis',(0.,-0.239315664287559,-0.970941817426052));
#55930=DIRECTION('center_axis',(-1.,0.,0.));
#55931=DIRECTION('ref_axis',(0.,0.,1.));
#55932=DIRECTION('center_axis',(0.,-0.88545602565321,0.464723172043769));
#55933=DIRECTION('ref_axis',(0.,-0.464723172043769,-0.88545602565321));
#55934=DIRECTION('center_axis',(0.,-0.748510748171101,0.663122658240796));
#55935=DIRECTION('ref_axis',(0.,-0.663122658240796,-0.748510748171101));
#55936=DIRECTION('center_axis',(0.,-0.568064746731156,0.822983865893657));
#55937=DIRECTION('ref_axis',(0.,-0.822983865893656,-0.568064746731156));
#55938=DIRECTION('center_axis',(0.,-0.354604887042536,0.935016242685415));
#55939=DIRECTION('ref_axis',(0.,-0.935016242685415,-0.354604887042536));
#55940=DIRECTION('center_axis',(0.,-0.120536680255322,0.992708874098054));
#55941=DIRECTION('ref_axis',(0.,-0.992708874098054,-0.120536680255322));
#55942=DIRECTION('center_axis',(0.,0.120536680255324,0.992708874098054));
#55943=DIRECTION('ref_axis',(0.,-0.992708874098054,0.120536680255324));
#55944=DIRECTION('center_axis',(0.,0.354604887042536,0.935016242685415));
#55945=DIRECTION('ref_axis',(0.,-0.935016242685415,0.354604887042536));
#55946=DIRECTION('center_axis',(0.,0.568064746731156,0.822983865893656));
#55947=DIRECTION('ref_axis',(0.,-0.822983865893656,0.568064746731156));
#55948=DIRECTION('center_axis',(0.,0.748510748171101,0.663122658240795));
#55949=DIRECTION('ref_axis',(0.,-0.663122658240795,0.748510748171101));
#55950=DIRECTION('center_axis',(0.,0.88545602565321,0.464723172043768));
#55951=DIRECTION('ref_axis',(0.,-0.464723172043768,0.88545602565321));
#55952=DIRECTION('center_axis',(0.,0.970941817426052,0.239315664287557));
#55953=DIRECTION('ref_axis',(0.,-0.239315664287557,0.970941817426052));
#55954=DIRECTION('center_axis',(0.,1.,-1.22464679914735E-16));
#55955=DIRECTION('ref_axis',(0.,1.22464679914735E-16,1.));
#55956=DIRECTION('center_axis',(0.,0.970941817426052,-0.239315664287558));
#55957=DIRECTION('ref_axis',(0.,0.239315664287558,0.970941817426052));
#55958=DIRECTION('center_axis',(0.,0.88545602565321,-0.464723172043769));
#55959=DIRECTION('ref_axis',(0.,0.464723172043769,0.88545602565321));
#55960=DIRECTION('center_axis',(0.,0.748510748171101,-0.663122658240796));
#55961=DIRECTION('ref_axis',(0.,0.663122658240796,0.748510748171101));
#55962=DIRECTION('center_axis',(0.,0.568064746731156,-0.822983865893656));
#55963=DIRECTION('ref_axis',(0.,0.822983865893656,0.568064746731156));
#55964=DIRECTION('center_axis',(0.,0.354604887042536,-0.935016242685415));
#55965=DIRECTION('ref_axis',(0.,0.935016242685415,0.354604887042536));
#55966=DIRECTION('center_axis',(0.,0.120536680255323,-0.992708874098054));
#55967=DIRECTION('ref_axis',(0.,0.992708874098054,0.120536680255323));
#55968=DIRECTION('center_axis',(0.,-0.120536680255323,-0.992708874098054));
#55969=DIRECTION('ref_axis',(0.,0.992708874098054,-0.120536680255323));
#55970=DIRECTION('center_axis',(0.,-0.354604887042536,-0.935016242685415));
#55971=DIRECTION('ref_axis',(0.,0.935016242685415,-0.354604887042536));
#55972=DIRECTION('center_axis',(0.,-0.568064746731156,-0.822983865893656));
#55973=DIRECTION('ref_axis',(0.,0.822983865893656,-0.568064746731156));
#55974=DIRECTION('center_axis',(0.,-0.748510748171101,-0.663122658240795));
#55975=DIRECTION('ref_axis',(0.,0.663122658240795,-0.748510748171101));
#55976=DIRECTION('center_axis',(0.,-0.88545602565321,-0.464723172043769));
#55977=DIRECTION('ref_axis',(0.,0.464723172043769,-0.88545602565321));
#55978=DIRECTION('center_axis',(0.,-0.970941817426052,-0.239315664287558));
#55979=DIRECTION('ref_axis',(0.,0.239315664287558,-0.970941817426052));
#55980=DIRECTION('center_axis',(1.,0.,0.));
#55981=DIRECTION('ref_axis',(0.,1.,0.));
#55982=DIRECTION('center_axis',(0.,-1.,0.));
#55983=DIRECTION('ref_axis',(0.,0.,-1.));
#55984=DIRECTION('center_axis',(1.,0.,0.));
#55985=DIRECTION('ref_axis',(0.,-0.5,-0.866025403784438));
#55986=DIRECTION('center_axis',(1.,0.,0.));
#55987=DIRECTION('ref_axis',(0.,-0.5,0.866025403784439));
#55988=DIRECTION('center_axis',(1.,0.,0.));
#55989=DIRECTION('ref_axis',(0.,0.,-1.));
#55990=DIRECTION('center_axis',(1.,0.,0.));
#55991=DIRECTION('ref_axis',(0.,0.866025403784439,0.5));
#55992=DIRECTION('center_axis',(1.,0.,0.));
#55993=DIRECTION('ref_axis',(0.,-0.499999999999999,0.866025403784439));
#55994=DIRECTION('center_axis',(-1.,0.,0.));
#55995=DIRECTION('ref_axis',(0.,1.,0.));
#55996=DIRECTION('',(-0.581238193719096,-0.813733471206735,-9.96536090872393E-17));
#55997=DIRECTION('center_axis',(-1.,0.,0.));
#55998=DIRECTION('ref_axis',(0.,0.,1.));
#86928=CARTESIAN_POINT('',(0.,0.,0.));
#86929=CARTESIAN_POINT('Origin',(613.,0.,0.));
#86930=CARTESIAN_POINT('',(614.,-1.95943487863577E-15,16.));
#86931=CARTESIAN_POINT('Origin',(614.,0.,0.));
#86932=CARTESIAN_POINT('',(613.,-2.0818995585505E-15,17.));
#86933=CARTESIAN_POINT('Origin',(613.,-1.95943487863577E-15,16.));
#86934=CARTESIAN_POINT('',(613.,-17.,-2.0818995585505E-15));
#86935=CARTESIAN_POINT('Origin',(613.,0.,0.));
#86936=CARTESIAN_POINT('Origin',(613.,0.,0.));
#86937=CARTESIAN_POINT('Origin',(609.,0.,0.));
#86938=CARTESIAN_POINT('',(604.,-17.,-2.0818995585505E-15));
#86939=CARTESIAN_POINT('',(609.,-17.,-2.0818995585505E-15));
#86940=CARTESIAN_POINT('Origin',(604.,0.,0.));
#86941=CARTESIAN_POINT('Origin',(614.,13.8,0.));
#86942=CARTESIAN_POINT('',(614.,-13.8,-1.69001258282335E-15));
#86943=CARTESIAN_POINT('Origin',(614.,0.,0.));
#86944=CARTESIAN_POINT('Origin',(603.,0.,0.));
#86945=CARTESIAN_POINT('',(604.,-2.20436423846524E-15,18.));
#86946=CARTESIAN_POINT('Origin',(604.,0.,0.));
#86947=CARTESIAN_POINT('',(603.,-2.32682891837997E-15,19.));
#86948=CARTESIAN_POINT('Origin',(603.,-2.20436423846524E-15,18.));
#86949=CARTESIAN_POINT('',(603.,-19.,-2.32682891837997E-15));
#86950=CARTESIAN_POINT('Origin',(603.,0.,0.));
#86951=CARTESIAN_POINT('Origin',(603.,0.,0.));
#86952=CARTESIAN_POINT('Origin',(595.,0.,0.));
#86953=CARTESIAN_POINT('',(586.,-19.,-2.32682891837997E-15));
#86954=CARTESIAN_POINT('',(595.,-19.,-2.32682891837997E-15));
#86955=CARTESIAN_POINT('Origin',(586.,0.,0.));
#86956=CARTESIAN_POINT('Origin',(604.,17.,0.));
#86957=CARTESIAN_POINT('Origin',(585.,0.,0.));
#86958=CARTESIAN_POINT('',(586.,-2.88389022669825E-15,23.548750780275));
#86959=CARTESIAN_POINT('Origin',(586.,0.,0.));
#86960=CARTESIAN_POINT('',(585.049937616944,-3.00620211219302E-15,24.5475031191528));
#86961=CARTESIAN_POINT('Origin',(585.,-2.88389022669825E-15,23.548750780275));
#86962=CARTESIAN_POINT('',(585.049937616944,-24.5475031191528,-3.00620211219302E-15));
#86963=CARTESIAN_POINT('Origin',(585.049937616944,0.,-3.75775264024127E-15));
#86964=CARTESIAN_POINT('Origin',(585.049937616944,0.,-3.75775264024127E-15));
#86965=CARTESIAN_POINT('Origin',(581.,0.,0.));
#86966=CARTESIAN_POINT('',(576.,-25.,-3.06161699786838E-15));
#86967=CARTESIAN_POINT('',(581.,-24.75,-3.0310008278897E-15));
#86968=CARTESIAN_POINT('Origin',(576.,0.,0.));
#86969=CARTESIAN_POINT('Origin',(586.,19.,0.));
#86970=CARTESIAN_POINT('Origin',(517.585786437627,0.,0.));
#86971=CARTESIAN_POINT('',(518.292893218813,-4.98518280221296E-15,40.7071067811865));
#86972=CARTESIAN_POINT('',(518.292893218813,-40.7071067811866,-4.98518280221296E-15));
#86973=CARTESIAN_POINT('Origin',(518.292893218813,0.,-6.2314785027662E-15));
#86974=CARTESIAN_POINT('Origin',(518.292893218813,0.,-6.2314785027662E-15));
#86975=CARTESIAN_POINT('',(517.585786437627,-5.02105187650415E-15,41.));
#86976=CARTESIAN_POINT('Origin',(517.585786437627,-4.89858719658941E-15,
40.));
#86977=CARTESIAN_POINT('',(517.585786437627,-41.,-5.02105187650415E-15));
#86978=CARTESIAN_POINT('Origin',(517.585786437627,0.,0.));
#86979=CARTESIAN_POINT('Origin',(517.585786437627,0.,0.));
#86980=CARTESIAN_POINT('Origin',(508.3,0.,0.));
#86981=CARTESIAN_POINT('',(499.014213562373,-41.,-5.02105187650415E-15));
#86982=CARTESIAN_POINT('',(508.3,-41.,-5.02105187650415E-15));
#86983=CARTESIAN_POINT('',(499.014213562373,-5.02105187650415E-15,41.));
#86984=CARTESIAN_POINT('Origin',(499.014213562373,0.,0.));
#86985=CARTESIAN_POINT('Origin',(499.014213562373,0.,0.));
#86986=CARTESIAN_POINT('Origin',(519.,0.,0.));
#86987=CARTESIAN_POINT('',(520.,6.16881793702417,38.5090338136371));
#86988=CARTESIAN_POINT('',(520.,-36.4342105263158,13.9121638620345));
#86989=CARTESIAN_POINT('Origin',(520.,0.,0.));
#86990=CARTESIAN_POINT('',(520.,30.2653925892916,24.5968699516026));
#86991=CARTESIAN_POINT('Origin',(520.,0.,0.));
#86992=CARTESIAN_POINT('',(520.,30.2653925892916,-24.5968699516026));
#86993=CARTESIAN_POINT('Origin',(520.,0.,0.));
#86994=CARTESIAN_POINT('',(520.,6.16881793702417,-38.5090338136371));
#86995=CARTESIAN_POINT('Origin',(520.,0.,0.));
#86996=CARTESIAN_POINT('',(520.,-36.4342105263158,-13.9121638620345));
#86997=CARTESIAN_POINT('Origin',(520.,0.,0.));
#86998=CARTESIAN_POINT('',(520.,-39.,-4.77612251667468E-15));
#86999=CARTESIAN_POINT('Origin',(520.,0.,0.));
#87000=CARTESIAN_POINT('',(519.,-40.,-4.89858719658941E-15));
#87001=CARTESIAN_POINT('Origin',(520.,0.,0.));
#87002=CARTESIAN_POINT('Origin',(499.014213562373,0.,0.));
#87003=CARTESIAN_POINT('',(498.307106781187,-4.98518280221296E-15,40.7071067811865));
#87004=CARTESIAN_POINT('Origin',(499.014213562373,-4.89858719658941E-15,
40.));
#87005=CARTESIAN_POINT('',(498.307106781187,-40.7071067811866,-4.98518280221297E-15));
#87006=CARTESIAN_POINT('Origin',(498.307106781187,0.,-6.2314785027662E-15));
#87007=CARTESIAN_POINT('Origin',(498.307106781187,0.,-6.2314785027662E-15));
#87008=CARTESIAN_POINT('Origin',(498.3,0.,0.));
#87009=CARTESIAN_POINT('',(498.292893218813,-40.6928932188135,-4.9834421428465E-15));
#87010=CARTESIAN_POINT('',(498.3,-40.7,-4.98431247252973E-15));
#87011=CARTESIAN_POINT('',(498.292893218813,-4.9834421428465E-15,40.6928932188135));
#87012=CARTESIAN_POINT('Origin',(498.292893218813,0.,-6.22930267855812E-15));
#87013=CARTESIAN_POINT('Origin',(498.292893218813,0.,-6.22930267855812E-15));
#87014=CARTESIAN_POINT('Origin',(524.5,5.99923847473991,18.0280098103812));
#87015=CARTESIAN_POINT('',(499.,4.99928462778598,18.0376173054777));
#87016=CARTESIAN_POINT('',(499.,5.68348908133255,17.0791671887822));
#87017=CARTESIAN_POINT('Origin',(499.,5.99923847473991,18.0280098103812));
#87018=CARTESIAN_POINT('',(552.,5.68348908133255,17.0791671887822));
#87019=CARTESIAN_POINT('',(524.5,5.68348908133255,17.0791671887822));
#87020=CARTESIAN_POINT('',(552.,4.99928462778598,18.0376173054777));
#87021=CARTESIAN_POINT('Origin',(552.,5.99923847473991,18.0280098103812));
#87022=CARTESIAN_POINT('',(524.5,4.99928462778598,18.0376173054777));
#87023=CARTESIAN_POINT('Origin',(499.,-10.5,18.1865334794732));
#87024=CARTESIAN_POINT('',(498.,5.99923847473991,18.0280098103812));
#87025=CARTESIAN_POINT('Origin',(499.,5.99923847473991,18.0280098103812));
#87026=CARTESIAN_POINT('',(499.,-18.1206771241785,4.68930116432717));
#87027=CARTESIAN_POINT('Origin',(499.,-10.5,18.1865334794732));
#87028=CARTESIAN_POINT('',(498.,-18.6123337128351,3.81851198270484));
#87029=CARTESIAN_POINT('Origin',(499.,-18.6123337128352,3.81851198270484));
#87030=CARTESIAN_POINT('Origin',(498.,-10.5,18.1865334794732));
#87031=CARTESIAN_POINT('Origin',(499.,5.99923847473991,18.0280098103812));
#87032=CARTESIAN_POINT('Origin',(499.,5.99923847473991,18.0280098103812));
#87033=CARTESIAN_POINT('Origin',(524.5,-18.6123337128351,3.81851198270483));
#87034=CARTESIAN_POINT('',(499.,-17.6327372016333,3.61753766782563));
#87035=CARTESIAN_POINT('Origin',(499.,-18.6123337128351,3.81851198270483));
#87036=CARTESIAN_POINT('',(552.,-18.1206771241785,4.68930116432716));
#87037=CARTESIAN_POINT('',(524.5,-18.1206771241785,4.68930116432716));
#87038=CARTESIAN_POINT('',(552.,-17.6327372016333,3.61753766782563));
#87039=CARTESIAN_POINT('Origin',(552.,-18.6123337128351,3.81851198270483));
#87040=CARTESIAN_POINT('',(524.5,-17.6327372016333,3.61753766782563));
#87041=CARTESIAN_POINT('Origin',(499.,-18.6123337128351,3.81851198270484));
#87042=CARTESIAN_POINT('Origin',(499.,-18.6123337128351,3.81851198270484));
#87043=CARTESIAN_POINT('Origin',(524.5,0.,0.));
#87044=CARTESIAN_POINT('',(499.,11.9492481203007,13.4616295209566));
#87045=CARTESIAN_POINT('Origin',(499.,0.,0.));
#87046=CARTESIAN_POINT('',(552.,11.9492481203008,13.4616295209566));
#87047=CARTESIAN_POINT('',(524.5,11.9492481203007,13.4616295209566));
#87048=CARTESIAN_POINT('Origin',(552.,0.,0.));
#87049=CARTESIAN_POINT('Origin',(499.,0.,0.));
#87050=CARTESIAN_POINT('',(498.,12.6130952380952,14.2094978276764));
#87051=CARTESIAN_POINT('Origin',(498.,0.,0.));
#87052=CARTESIAN_POINT('Origin',(499.,12.6130952380952,14.2094978276764));
#87053=CARTESIAN_POINT('Origin',(498.,40.4,0.));
#87054=CARTESIAN_POINT('',(498.,-4.89684653722295E-15,39.9857864376269));
#87055=CARTESIAN_POINT('Origin',(498.,0.,0.));
#87056=CARTESIAN_POINT('',(498.,-18.6123337128351,-3.81851198270482));
#87057=CARTESIAN_POINT('Origin',(498.,0.,0.));
#87058=CARTESIAN_POINT('',(498.,5.9992384747399,-18.0280098103812));
#87059=CARTESIAN_POINT('Origin',(498.,-10.5,-18.1865334794732));
#87060=CARTESIAN_POINT('',(498.,12.6130952380952,-14.2094978276764));
#87061=CARTESIAN_POINT('Origin',(498.,0.,0.));
#87062=CARTESIAN_POINT('Origin',(498.,21.,0.));
#87063=CARTESIAN_POINT('Origin',(499.,0.,0.));
#87064=CARTESIAN_POINT('',(499.,-17.6327372016333,-3.61753766782562));
#87065=CARTESIAN_POINT('Origin',(499.,0.,0.));
#87066=CARTESIAN_POINT('Origin',(499.,-18.6123337128351,-3.81851198270482));
#87067=CARTESIAN_POINT('Origin',(524.5,0.,0.));
#87068=CARTESIAN_POINT('',(552.,-17.6327372016333,-3.61753766782562));
#87069=CARTESIAN_POINT('Origin',(552.,0.,0.));
#87070=CARTESIAN_POINT('',(524.5,-17.6327372016333,-3.61753766782562));
#87071=CARTESIAN_POINT('Origin',(524.5,12.6130952380952,14.2094978276764));
#87072=CARTESIAN_POINT('',(499.,13.1213924963925,13.3483161411505));
#87073=CARTESIAN_POINT('Origin',(499.,12.6130952380952,14.2094978276764));
#87074=CARTESIAN_POINT('',(552.,13.1213924963925,13.3483161411505));
#87075=CARTESIAN_POINT('',(524.5,13.1213924963925,13.3483161411505));
#87076=CARTESIAN_POINT('Origin',(552.,12.6130952380952,14.2094978276764));
#87077=CARTESIAN_POINT('Origin',(499.,12.6130952380952,14.2094978276764));
#87078=CARTESIAN_POINT('Origin',(499.,12.6130952380952,14.2094978276764));
#87079=CARTESIAN_POINT('Origin',(497.,21.,0.));
#87080=CARTESIAN_POINT('',(499.,13.1213924963925,-13.3483161411505));
#87081=CARTESIAN_POINT('Origin',(499.,21.,0.));
#87082=CARTESIAN_POINT('',(552.,13.1213924963925,-13.3483161411505));
#87083=CARTESIAN_POINT('',(524.5,13.1213924963925,-13.3483161411505));
#87084=CARTESIAN_POINT('Origin',(552.,21.,0.));
#87085=CARTESIAN_POINT('Origin',(499.,21.,0.));
#87086=CARTESIAN_POINT('Origin',(499.,12.6130952380952,-14.2094978276764));
#87087=CARTESIAN_POINT('Origin',(499.,0.,0.));
#87088=CARTESIAN_POINT('Origin',(499.,-4.89684653722295E-15,39.9857864376269));
#87089=CARTESIAN_POINT('Origin',(543.,-35.5,-13.555441711726));
#87090=CARTESIAN_POINT('',(520.352412817281,-36.5,-13.5554416839856));
#87091=CARTESIAN_POINT('Ctrl Pts',(520.,-36.4342105263158,-13.9121638620345));
#87092=CARTESIAN_POINT('Ctrl Pts',(520.001409159077,-36.4347197758084,-13.9108302015481));
#87093=CARTESIAN_POINT('Ctrl Pts',(520.002818319607,-36.4352261699646,-13.9094954491959));
#87094=CARTESIAN_POINT('Ctrl Pts',(520.106030195301,-36.472107069984,-13.8116536513495));
#87095=CARTESIAN_POINT('Ctrl Pts',(520.208354938718,-36.4937643512708,-13.7089641296516));
#87096=CARTESIAN_POINT('Ctrl Pts',(520.322544608623,-36.499610188676,-13.5876050900205));
#87097=CARTESIAN_POINT('Ctrl Pts',(520.337509666305,-36.5000000006532,-13.571561539651));
#87098=CARTESIAN_POINT('Ctrl Pts',(520.352412803453,-36.5,-13.5554416712017));
#87099=CARTESIAN_POINT('',(566.,-36.4342105263158,-13.9121638620345));
#87100=CARTESIAN_POINT('',(543.,-36.4342105263158,-13.9121638620345));
#87101=CARTESIAN_POINT('',(565.647587182719,-36.5,-13.5554416839856));
#87102=CARTESIAN_POINT('Ctrl Pts',(565.647587196547,-36.5,-13.5554416712016));
#87103=CARTESIAN_POINT('Ctrl Pts',(565.662490333695,-36.5000000006532,-13.5715615396511));
#87104=CARTESIAN_POINT('Ctrl Pts',(565.677455391377,-36.4996101886759,-13.5876050900207));
#87105=CARTESIAN_POINT('Ctrl Pts',(565.791645061283,-36.4937643512707,-13.7089641296523));
#87106=CARTESIAN_POINT('Ctrl Pts',(565.893969804688,-36.4721070699799,-13.8116536513606));
#87107=CARTESIAN_POINT('Ctrl Pts',(565.997181680394,-36.4352261699646,-13.9094954491958));
#87108=CARTESIAN_POINT('Ctrl Pts',(565.998590840923,-36.4347197758083,-13.9108302015484));
#87109=CARTESIAN_POINT('Ctrl Pts',(566.,-36.4342105263158,-13.9121638620345));
#87110=CARTESIAN_POINT('',(543.,-36.5,-13.555441711726));
#87111=CARTESIAN_POINT('Origin',(565.,-36.5,0.));
#87112=CARTESIAN_POINT('',(565.,-36.5,-10.571187255933));
#87113=CARTESIAN_POINT('Ctrl Pts',(565.647587196547,-36.5,-13.5554416712018));
#87114=CARTESIAN_POINT('Ctrl Pts',(565.568128153195,-36.5,-13.4694953732581));
#87115=CARTESIAN_POINT('Ctrl Pts',(565.501742890333,-36.5,-13.3629845948168));
#87116=CARTESIAN_POINT('Ctrl Pts',(565.249597405087,-36.5,-12.8781277023248));
#87117=CARTESIAN_POINT('Ctrl Pts',(565.151696115369,-36.5,-12.4208012195937));
#87118=CARTESIAN_POINT('Ctrl Pts',(565.021905737199,-36.5,-11.4862782354435));
#87119=CARTESIAN_POINT('Ctrl Pts',(565.,-36.5,-11.0077223622835));
#87120=CARTESIAN_POINT('Ctrl Pts',(565.,-36.5,-10.5711872559327));
#87121=CARTESIAN_POINT('',(565.,-36.5,10.571187255933));
#87122=CARTESIAN_POINT('',(565.,-36.5,0.));
#87123=CARTESIAN_POINT('',(565.647587182719,-36.5,13.5554416839856));
#87124=CARTESIAN_POINT('Ctrl Pts',(565.,-36.5,10.5711872559327));
#87125=CARTESIAN_POINT('Ctrl Pts',(565.,-36.5,11.0077223622835));
#87126=CARTESIAN_POINT('Ctrl Pts',(565.021905737199,-36.5,11.4862782354435));
#87127=CARTESIAN_POINT('Ctrl Pts',(565.151696115369,-36.5,12.4208012195937));
#87128=CARTESIAN_POINT('Ctrl Pts',(565.249597405087,-36.5,12.8781277023248));
#87129=CARTESIAN_POINT('Ctrl Pts',(565.501742890333,-36.5,13.3629845948168));
#87130=CARTESIAN_POINT('Ctrl Pts',(565.568128153195,-36.5,13.469495373258));
#87131=CARTESIAN_POINT('Ctrl Pts',(565.647587196547,-36.5,13.5554416712017));
#87132=CARTESIAN_POINT('',(520.352412817281,-36.5,13.5554416839856));
#87133=CARTESIAN_POINT('',(543.,-36.5,13.555441711726));
#87134=CARTESIAN_POINT('',(521.,-36.5,10.571187255933));
#87135=CARTESIAN_POINT('Ctrl Pts',(520.352412803453,-36.5,13.5554416712018));
#87136=CARTESIAN_POINT('Ctrl Pts',(520.431871846805,-36.5,13.4694953732582));
#87137=CARTESIAN_POINT('Ctrl Pts',(520.498257109667,-36.5,13.3629845948169));
#87138=CARTESIAN_POINT('Ctrl Pts',(520.750402594913,-36.5,12.878127702325));
#87139=CARTESIAN_POINT('Ctrl Pts',(520.848303884631,-36.5,12.4208012195939));
#87140=CARTESIAN_POINT('Ctrl Pts',(520.978094262801,-36.5,11.4862782354437));
#87141=CARTESIAN_POINT('Ctrl Pts',(521.,-36.5,11.0077223622837));
#87142=CARTESIAN_POINT('Ctrl Pts',(521.,-36.5,10.571187255933));
#87143=CARTESIAN_POINT('',(521.,-36.5,-10.571187255933));
#87144=CARTESIAN_POINT('',(521.,-36.5,0.));
#87145=CARTESIAN_POINT('Ctrl Pts',(521.,-36.5,-10.571187255933));
#87146=CARTESIAN_POINT('Ctrl Pts',(521.,-36.5,-11.0077223622837));
#87147=CARTESIAN_POINT('Ctrl Pts',(520.978094262801,-36.5,-11.4862782354437));
#87148=CARTESIAN_POINT('Ctrl Pts',(520.848303884631,-36.5,-12.4208012195939));
#87149=CARTESIAN_POINT('Ctrl Pts',(520.750402594913,-36.5,-12.878127702325));
#87150=CARTESIAN_POINT('Ctrl Pts',(520.498257109667,-36.5,-13.3629845948169));
#87151=CARTESIAN_POINT('Ctrl Pts',(520.431871846805,-36.5,-13.4694953732582));
#87152=CARTESIAN_POINT('Ctrl Pts',(520.352412803453,-36.5,-13.5554416712018));
#87153=CARTESIAN_POINT('Origin',(543.,-35.5,13.555441711726));
#87154=CARTESIAN_POINT('',(566.,-36.4342105263158,13.9121638620345));
#87155=CARTESIAN_POINT('Ctrl Pts',(566.,-36.4342105263158,13.9121638620345));
#87156=CARTESIAN_POINT('Ctrl Pts',(565.998590840923,-36.4347197758084,13.9108302015481));
#87157=CARTESIAN_POINT('Ctrl Pts',(565.997181680393,-36.4352261699646,13.9094954491959));
#87158=CARTESIAN_POINT('Ctrl Pts',(565.893969804699,-36.472107069984,13.8116536513495));
#87159=CARTESIAN_POINT('Ctrl Pts',(565.791645061282,-36.4937643512708,13.7089641296516));
#87160=CARTESIAN_POINT('Ctrl Pts',(565.677455391377,-36.499610188676,13.5876050900205));
#87161=CARTESIAN_POINT('Ctrl Pts',(565.662490333695,-36.5000000006532,13.571561539651));
#87162=CARTESIAN_POINT('Ctrl Pts',(565.647587196547,-36.5,13.5554416712017));
#87163=CARTESIAN_POINT('',(543.,-36.4342105263158,13.9121638620345));
#87164=CARTESIAN_POINT('Ctrl Pts',(520.352412803453,-36.5,13.5554416712017));
#87165=CARTESIAN_POINT('Ctrl Pts',(520.337509666304,-36.5000000006532,13.5715615396511));
#87166=CARTESIAN_POINT('Ctrl Pts',(520.322544608623,-36.4996101886759,13.5876050900207));
#87167=CARTESIAN_POINT('Ctrl Pts',(520.208354938717,-36.4937643512707,13.7089641296523));
#87168=CARTESIAN_POINT('Ctrl Pts',(520.106030195312,-36.4721070699799,13.8116536513606));
#87169=CARTESIAN_POINT('Ctrl Pts',(520.002818319606,-36.4352261699646,13.9094954491959));
#87170=CARTESIAN_POINT('Ctrl Pts',(520.001409159077,-36.4347197758083,13.9108302015484));
#87171=CARTESIAN_POINT('Ctrl Pts',(520.,-36.4342105263158,13.9121638620345));
#87172=CARTESIAN_POINT('Origin',(524.5,-18.6123337128351,-3.81851198270482));
#87173=CARTESIAN_POINT('',(499.,-18.1206771241785,-4.68930116432715));
#87174=CARTESIAN_POINT('Origin',(499.,-18.6123337128351,-3.81851198270482));
#87175=CARTESIAN_POINT('',(552.,-18.1206771241785,-4.68930116432715));
#87176=CARTESIAN_POINT('Origin',(552.,-18.6123337128351,-3.81851198270482));
#87177=CARTESIAN_POINT('',(524.5,-18.1206771241785,-4.68930116432715));
#87178=CARTESIAN_POINT('Origin',(499.,-18.6123337128351,-3.81851198270482));
#87179=CARTESIAN_POINT('Origin',(499.,-18.6123337128351,-3.81851198270482));
#87180=CARTESIAN_POINT('Origin',(499.,-10.5,-18.1865334794732));
#87181=CARTESIAN_POINT('',(499.,4.99928462778596,-18.0376173054777));
#87182=CARTESIAN_POINT('Origin',(499.,-10.5,-18.1865334794732));
#87183=CARTESIAN_POINT('Origin',(499.,5.9992384747399,-18.0280098103812));
#87184=CARTESIAN_POINT('Origin',(497.,-10.5,-18.1865334794732));
#87185=CARTESIAN_POINT('',(552.,4.99928462778596,-18.0376173054777));
#87186=CARTESIAN_POINT('Origin',(552.,-10.5,-18.1865334794732));
#87187=CARTESIAN_POINT('',(524.5,4.99928462778596,-18.0376173054777));
#87188=CARTESIAN_POINT('Origin',(524.5,12.6130952380952,-14.2094978276764));
#87189=CARTESIAN_POINT('',(499.,11.9492481203008,-13.4616295209566));
#87190=CARTESIAN_POINT('Origin',(499.,12.6130952380952,-14.2094978276764));
#87191=CARTESIAN_POINT('',(552.,11.9492481203008,-13.4616295209566));
#87192=CARTESIAN_POINT('',(524.5,11.9492481203008,-13.4616295209566));
#87193=CARTESIAN_POINT('Origin',(552.,12.6130952380952,-14.2094978276764));
#87194=CARTESIAN_POINT('Origin',(499.,12.6130952380952,-14.2094978276764));
#87195=CARTESIAN_POINT('Origin',(499.,12.6130952380952,-14.2094978276764));
#87196=CARTESIAN_POINT('Origin',(499.,0.,0.));
#87197=CARTESIAN_POINT('',(499.,5.68348908133254,-17.0791671887822));
#87198=CARTESIAN_POINT('Origin',(499.,5.9992384747399,-18.0280098103812));
#87199=CARTESIAN_POINT('Origin',(499.,0.,0.));
#87200=CARTESIAN_POINT('Origin',(499.,5.9992384747399,-18.0280098103812));
#87201=CARTESIAN_POINT('Origin',(499.,5.9992384747399,-18.0280098103812));
#87202=CARTESIAN_POINT('Origin',(524.5,0.,0.));
#87203=CARTESIAN_POINT('',(552.,5.68348908133254,-17.0791671887822));
#87204=CARTESIAN_POINT('',(524.5,5.68348908133254,-17.0791671887822));
#87205=CARTESIAN_POINT('Origin',(552.,0.,0.));
#87206=CARTESIAN_POINT('Origin',(524.5,5.9992384747399,-18.0280098103812));
#87207=CARTESIAN_POINT('Origin',(552.,5.9992384747399,-18.0280098103812));
#87208=CARTESIAN_POINT('Origin',(566.,0.,0.));
#87209=CARTESIAN_POINT('Origin',(565.,0.,0.));
#87210=CARTESIAN_POINT('',(566.,-39.,-4.77612251667468E-15));
#87211=CARTESIAN_POINT('Origin',(566.,0.,0.));
#87212=CARTESIAN_POINT('Origin',(566.,0.,0.));
#87213=CARTESIAN_POINT('Origin',(565.,-45.,0.));
#87214=CARTESIAN_POINT('Origin',(543.,0.,0.));
#87215=CARTESIAN_POINT('',(566.,6.16881793702417,38.5090338136371));
#87216=CARTESIAN_POINT('Origin',(566.,0.,0.));
#87217=CARTESIAN_POINT('',(543.,6.16881793702417,38.5090338136371));
#87218=CARTESIAN_POINT('Origin',(520.,0.,0.));
#87219=CARTESIAN_POINT('Origin',(521.,0.,0.));
#87220=CARTESIAN_POINT('Origin',(521.,-36.5,0.));
#87221=CARTESIAN_POINT('Origin',(520.,0.,0.));
#87222=CARTESIAN_POINT('',(520.352412765988,29.9893568818739,-24.832206382269));
#87223=CARTESIAN_POINT('Ctrl Pts',(520.,30.2653925892916,-24.5968699516026));
#87224=CARTESIAN_POINT('Ctrl Pts',(520.00149020625,30.2644404464129,-24.5980415225416));
#87225=CARTESIAN_POINT('Ctrl Pts',(520.002980414215,30.2634856493794,-24.5992109386738));
#87226=CARTESIAN_POINT('Ctrl Pts',(520.108399039101,30.1957548087309,-24.6817839028605));
#87227=CARTESIAN_POINT('Ctrl Pts',(520.212881902993,30.1157230092887,-24.7531338324709));
#87228=CARTESIAN_POINT('Ctrl Pts',(520.326848640886,30.0130697413226,-24.8181858293159));
#87229=CARTESIAN_POINT('Ctrl Pts',(520.339653361077,30.0013089989909,-24.8253058242341));
#87230=CARTESIAN_POINT('Ctrl Pts',(520.352412765988,29.9893568818739,-24.832206382269));
#87231=CARTESIAN_POINT('',(521.,27.4049167118003,-26.3243336101655));
#87232=CARTESIAN_POINT('Ctrl Pts',(520.352412765988,29.9893568818739,-24.8322063822691));
#87233=CARTESIAN_POINT('Ctrl Pts',(520.431871825795,29.9149251983096,-24.8751795348111));
#87234=CARTESIAN_POINT('Ctrl Pts',(520.498257101696,29.8226841427655,-24.9284349330598));
#87235=CARTESIAN_POINT('Ctrl Pts',(520.750402594913,29.4027857433936,-25.1708633869695));
#87236=CARTESIAN_POINT('Ctrl Pts',(520.848303884631,29.006729391525,-25.3995266283351));
#87237=CARTESIAN_POINT('Ctrl Pts',(520.978094262801,28.1974087468305,-25.8667881204102));
#87238=CARTESIAN_POINT('Ctrl Pts',(521.,27.7829672035437,-26.1060660569902));
#87239=CARTESIAN_POINT('Ctrl Pts',(521.,27.4049167118003,-26.3243336101655));
#87240=CARTESIAN_POINT('',(521.,9.09508328819973,-36.8955208660985));
#87241=CARTESIAN_POINT('Origin',(521.,0.,0.));
#87242=CARTESIAN_POINT('',(520.352412765988,6.51064311812611,-38.387648093995));
#87243=CARTESIAN_POINT('Ctrl Pts',(521.,9.09508328819973,-36.8955208660985));
#87244=CARTESIAN_POINT('Ctrl Pts',(521.,8.71703279645624,-37.1137884192739));
#87245=CARTESIAN_POINT('Ctrl Pts',(520.978094262801,8.30259125316945,-37.3530663558539));
#87246=CARTESIAN_POINT('Ctrl Pts',(520.848303884631,7.49327060847496,-37.820327847929));
#87247=CARTESIAN_POINT('Ctrl Pts',(520.750402594913,7.09721425660644,-38.0489910892945));
#87248=CARTESIAN_POINT('Ctrl Pts',(520.498257101696,6.67731585723445,-38.2914195432042));
#87249=CARTESIAN_POINT('Ctrl Pts',(520.431871825795,6.58507480169031,-38.344674941453));
#87250=CARTESIAN_POINT('Ctrl Pts',(520.352412765988,6.5106431181261,-38.387648093995));
#87251=CARTESIAN_POINT('Ctrl Pts',(520.352412765988,6.51064311812611,-38.387648093995));
#87252=CARTESIAN_POINT('Ctrl Pts',(520.239409874431,6.40478992169232,-38.4487624654506));
#87253=CARTESIAN_POINT('Ctrl Pts',(520.12154020013,6.29031027699351,-38.4890173932814));
#87254=CARTESIAN_POINT('Ctrl Pts',(520.002980414215,6.17179876125379,-38.5085528487653));
#87255=CARTESIAN_POINT('Ctrl Pts',(520.001490206249,6.17030861865822,-38.5087950191858));
#87256=CARTESIAN_POINT('Ctrl Pts',(520.,6.16881793702417,-38.5090338136371));
#87257=CARTESIAN_POINT('Origin',(543.,29.4893568818739,-23.9661809784846));
#87258=CARTESIAN_POINT('',(565.647587234012,29.9893568818739,-24.832206382269));
#87259=CARTESIAN_POINT('',(543.,29.9893568818739,-24.832206382269));
#87260=CARTESIAN_POINT('',(566.,30.2653925892916,-24.5968699516026));
#87261=CARTESIAN_POINT('',(543.,30.2653925892916,-24.5968699516026));
#87262=CARTESIAN_POINT('Ctrl Pts',(566.,30.2653925892916,-24.5968699516026));
#87263=CARTESIAN_POINT('Ctrl Pts',(565.99850979375,30.2644404464129,-24.5980415225416));
#87264=CARTESIAN_POINT('Ctrl Pts',(565.997019585785,30.2634856493794,-24.5992109386738));
#87265=CARTESIAN_POINT('Ctrl Pts',(565.891600960899,30.1957548087313,-24.6817839028601));
#87266=CARTESIAN_POINT('Ctrl Pts',(565.787118097009,30.1157230092896,-24.7531338324701));
#87267=CARTESIAN_POINT('Ctrl Pts',(565.673151359116,30.0130697413237,-24.8181858293152));
#87268=CARTESIAN_POINT('Ctrl Pts',(565.660346638924,30.0013089989915,-24.8253058242338));
#87269=CARTESIAN_POINT('Ctrl Pts',(565.647587234012,29.9893568818739,-24.8322063822691));
#87270=CARTESIAN_POINT('Origin',(543.,6.01064311812611,-37.5216226902105));
#87271=CARTESIAN_POINT('',(565.647587234012,6.51064311812611,-38.387648093995));
#87272=CARTESIAN_POINT('',(543.,6.51064311812611,-38.387648093995));
#87273=CARTESIAN_POINT('',(566.,6.16881793702416,-38.5090338136371));
#87274=CARTESIAN_POINT('Ctrl Pts',(565.647587234012,6.51064311812611,-38.387648093995));
#87275=CARTESIAN_POINT('Ctrl Pts',(565.760590125569,6.4047899216923,-38.4487624654506));
#87276=CARTESIAN_POINT('Ctrl Pts',(565.878459799869,6.29031027699293,-38.4890173932815));
#87277=CARTESIAN_POINT('Ctrl Pts',(565.997019585785,6.17179876125356,-38.5085528487653));
#87278=CARTESIAN_POINT('Ctrl Pts',(565.998509793751,6.17030861865838,-38.5087950191857));
#87279=CARTESIAN_POINT('Ctrl Pts',(566.,6.16881793702416,-38.5090338136371));
#87280=CARTESIAN_POINT('',(543.,6.16881793702416,-38.5090338136371));
#87281=CARTESIAN_POINT('Origin',(566.,0.,0.));
#87282=CARTESIAN_POINT('Origin',(566.,0.,0.));
#87283=CARTESIAN_POINT('',(565.,9.09508328819973,-36.8955208660985));
#87284=CARTESIAN_POINT('Ctrl Pts',(565.647587234012,6.51064311812611,-38.387648093995));
#87285=CARTESIAN_POINT('Ctrl Pts',(565.568128174205,6.58507480169041,-38.3446749414529));
#87286=CARTESIAN_POINT('Ctrl Pts',(565.501742898304,6.67731585723452,-38.2914195432042));
#87287=CARTESIAN_POINT('Ctrl Pts',(565.249597405087,7.09721425660658,-38.0489910892944));
#87288=CARTESIAN_POINT('Ctrl Pts',(565.151696115369,7.49327060847513,-37.8203278479289));
#87289=CARTESIAN_POINT('Ctrl Pts',(565.0219057372,8.30259125316967,-37.3530663558537));
#87290=CARTESIAN_POINT('Ctrl Pts',(565.,8.71703279645644,-37.1137884192738));
#87291=CARTESIAN_POINT('Ctrl Pts',(565.,9.09508328819994,-36.8955208660984));
#87292=CARTESIAN_POINT('',(565.,27.4049167118003,-26.3243336101655));
#87293=CARTESIAN_POINT('Origin',(565.,0.,0.));
#87294=CARTESIAN_POINT('Ctrl Pts',(565.,27.4049167118001,-26.3243336101657));
#87295=CARTESIAN_POINT('Ctrl Pts',(565.,27.7829672035435,-26.1060660569903));
#87296=CARTESIAN_POINT('Ctrl Pts',(565.021905737199,28.1974087468303,-25.8667881204103));
#87297=CARTESIAN_POINT('Ctrl Pts',(565.151696115369,29.0067293915249,-25.3995266283352));
#87298=CARTESIAN_POINT('Ctrl Pts',(565.249597405087,29.4027857433934,-25.1708633869696));
#87299=CARTESIAN_POINT('Ctrl Pts',(565.501742898304,29.8226841427655,-24.9284349330599));
#87300=CARTESIAN_POINT('Ctrl Pts',(565.568128174205,29.9149251983096,-24.8751795348111));
#87301=CARTESIAN_POINT('Ctrl Pts',(565.647587234012,29.9893568818739,-24.8322063822691));
#87302=CARTESIAN_POINT('Origin',(565.,18.25,-31.609927238132));
#87303=CARTESIAN_POINT('',(521.,18.25,-31.609927238132));
#87304=CARTESIAN_POINT('',(565.,18.25,-31.609927238132));
#87305=CARTESIAN_POINT('Origin',(521.,18.25,-31.609927238132));
#87306=CARTESIAN_POINT('Origin',(543.,0.,0.));
#87307=CARTESIAN_POINT('Origin',(566.,0.,0.));
#87308=CARTESIAN_POINT('Origin',(543.,0.,0.));
#87309=CARTESIAN_POINT('',(566.,30.2653925892916,24.5968699516026));
#87310=CARTESIAN_POINT('',(543.,30.2653925892916,24.5968699516026));
#87311=CARTESIAN_POINT('Origin',(566.,0.,0.));
#87312=CARTESIAN_POINT('Origin',(520.,0.,0.));
#87313=CARTESIAN_POINT('',(520.352412765988,6.51064311812612,38.387648093995));
#87314=CARTESIAN_POINT('Ctrl Pts',(520.,6.16881793702417,38.5090338136371));
#87315=CARTESIAN_POINT('Ctrl Pts',(520.00149020625,6.17030861865913,38.5087950191856));
#87316=CARTESIAN_POINT('Ctrl Pts',(520.002980414216,6.1717987612548,38.5085528487651));
#87317=CARTESIAN_POINT('Ctrl Pts',(520.108399039102,6.27717446622854,38.4911827022374));
#87318=CARTESIAN_POINT('Ctrl Pts',(520.212881902991,6.37898121755002,38.4575480956155));
#87319=CARTESIAN_POINT('Ctrl Pts',(520.326848640884,6.48664453336754,38.4011737561983));
#87320=CARTESIAN_POINT('Ctrl Pts',(520.339653361076,6.49869100100822,38.3945486520304));
#87321=CARTESIAN_POINT('Ctrl Pts',(520.352412765988,6.51064311812613,38.387648093995));
#87322=CARTESIAN_POINT('',(521.,9.09508328819974,36.8955208660985));
#87323=CARTESIAN_POINT('Ctrl Pts',(520.352412765988,6.51064311812613,38.387648093995));
#87324=CARTESIAN_POINT('Ctrl Pts',(520.431871825795,6.58507480169035,38.3446749414529));
#87325=CARTESIAN_POINT('Ctrl Pts',(520.498257101696,6.67731585723446,38.2914195432042));
#87326=CARTESIAN_POINT('Ctrl Pts',(520.750402594913,7.09721425660646,38.0489910892945));
#87327=CARTESIAN_POINT('Ctrl Pts',(520.848303884631,7.49327060847499,37.8203278479289));
#87328=CARTESIAN_POINT('Ctrl Pts',(520.978094262801,8.30259125316947,37.3530663558539));
#87329=CARTESIAN_POINT('Ctrl Pts',(521.,8.71703279645626,37.1137884192739));
#87330=CARTESIAN_POINT('Ctrl Pts',(521.,9.09508328819974,36.8955208660985));
#87331=CARTESIAN_POINT('',(521.,27.4049167118003,26.3243336101655));
#87332=CARTESIAN_POINT('Origin',(521.,0.,0.));
#87333=CARTESIAN_POINT('',(520.352412765988,29.9893568818739,24.832206382269));
#87334=CARTESIAN_POINT('Ctrl Pts',(521.,27.4049167118003,26.3243336101655));
#87335=CARTESIAN_POINT('Ctrl Pts',(521.,27.7829672035438,26.1060660569901));
#87336=CARTESIAN_POINT('Ctrl Pts',(520.978094262801,28.1974087468306,25.8667881204101));
#87337=CARTESIAN_POINT('Ctrl Pts',(520.848303884631,29.006729391525,25.3995266283351));
#87338=CARTESIAN_POINT('Ctrl Pts',(520.750402594913,29.4027857433936,25.1708633869695));
#87339=CARTESIAN_POINT('Ctrl Pts',(520.498257101696,29.8226841427656,24.9284349330598));
#87340=CARTESIAN_POINT('Ctrl Pts',(520.431871825795,29.9149251983096,24.8751795348111));
#87341=CARTESIAN_POINT('Ctrl Pts',(520.352412765988,29.9893568818739,24.832206382269));
#87342=CARTESIAN_POINT('Ctrl Pts',(520.352412765988,29.9893568818739,24.832206382269));
#87343=CARTESIAN_POINT('Ctrl Pts',(520.239409874432,30.0952100783073,24.7710920108136));
#87344=CARTESIAN_POINT('Ctrl Pts',(520.121540200111,30.187311690774,24.6920771942183));
#87345=CARTESIAN_POINT('Ctrl Pts',(520.002980414217,30.2634856493798,24.5992109386733));
#87346=CARTESIAN_POINT('Ctrl Pts',(520.001490206249,30.2644404464136,24.5980415225407));
#87347=CARTESIAN_POINT('Ctrl Pts',(520.,30.2653925892916,24.5968699516026));
#87348=CARTESIAN_POINT('Origin',(543.,6.01064311812612,37.5216226902105));
#87349=CARTESIAN_POINT('',(565.647587234012,6.51064311812612,38.387648093995));
#87350=CARTESIAN_POINT('',(543.,6.51064311812612,38.387648093995));
#87351=CARTESIAN_POINT('Ctrl Pts',(566.,6.16881793702417,38.5090338136371));
#87352=CARTESIAN_POINT('Ctrl Pts',(565.99850979375,6.17030861865904,38.5087950191856));
#87353=CARTESIAN_POINT('Ctrl Pts',(565.997019585784,6.17179876125457,38.5085528487651));
#87354=CARTESIAN_POINT('Ctrl Pts',(565.891600960899,6.27717446622842,38.4911827022375));
#87355=CARTESIAN_POINT('Ctrl Pts',(565.787118097009,6.37898121754967,38.4575480956156));
#87356=CARTESIAN_POINT('Ctrl Pts',(565.673151359116,6.48664453336733,38.4011737561984));
#87357=CARTESIAN_POINT('Ctrl Pts',(565.660346638924,6.49869100100812,38.3945486520304));
#87358=CARTESIAN_POINT('Ctrl Pts',(565.647587234012,6.51064311812612,38.387648093995));
#87359=CARTESIAN_POINT('Origin',(543.,29.4893568818739,23.9661809784846));
#87360=CARTESIAN_POINT('',(565.647587234012,29.9893568818739,24.832206382269));
#87361=CARTESIAN_POINT('',(543.,29.9893568818739,24.832206382269));
#87362=CARTESIAN_POINT('Ctrl Pts',(565.647587234012,29.9893568818739,24.832206382269));
#87363=CARTESIAN_POINT('Ctrl Pts',(565.760590125568,30.0952100783073,24.7710920108136));
#87364=CARTESIAN_POINT('Ctrl Pts',(565.878459799889,30.1873116907738,24.6920771942186));
#87365=CARTESIAN_POINT('Ctrl Pts',(565.997019585783,30.2634856493799,24.5992109386732));
#87366=CARTESIAN_POINT('Ctrl Pts',(565.998509793751,30.2644404464136,24.5980415225408));
#87367=CARTESIAN_POINT('Ctrl Pts',(566.,30.2653925892916,24.5968699516026));
#87368=CARTESIAN_POINT('Origin',(566.,0.,0.));
#87369=CARTESIAN_POINT('Origin',(566.,0.,0.));
#87370=CARTESIAN_POINT('',(565.,27.4049167118003,26.3243336101655));
#87371=CARTESIAN_POINT('Ctrl Pts',(565.647587234012,29.9893568818739,24.832206382269));
#87372=CARTESIAN_POINT('Ctrl Pts',(565.568128174205,29.9149251983096,24.8751795348111));
#87373=CARTESIAN_POINT('Ctrl Pts',(565.501742898304,29.8226841427655,24.9284349330598));
#87374=CARTESIAN_POINT('Ctrl Pts',(565.249597405087,29.4027857433934,25.1708633869696));
#87375=CARTESIAN_POINT('Ctrl Pts',(565.151696115369,29.0067293915249,25.3995266283352));
#87376=CARTESIAN_POINT('Ctrl Pts',(565.021905737199,28.1974087468303,25.8667881204103));
#87377=CARTESIAN_POINT('Ctrl Pts',(565.,27.7829672035436,26.1060660569903));
#87378=CARTESIAN_POINT('Ctrl Pts',(565.,27.4049167118001,26.3243336101656));
#87379=CARTESIAN_POINT('',(565.,9.09508328819974,36.8955208660985));
#87380=CARTESIAN_POINT('Origin',(565.,0.,0.));
#87381=CARTESIAN_POINT('Ctrl Pts',(565.,9.09508328819997,36.8955208660984));
#87382=CARTESIAN_POINT('Ctrl Pts',(565.,8.71703279645647,37.1137884192737));
#87383=CARTESIAN_POINT('Ctrl Pts',(565.021905737199,8.30259125316969,37.3530663558537));
#87384=CARTESIAN_POINT('Ctrl Pts',(565.151696115369,7.49327060847515,37.8203278479289));
#87385=CARTESIAN_POINT('Ctrl Pts',(565.249597405087,7.09721425660661,38.0489910892944));
#87386=CARTESIAN_POINT('Ctrl Pts',(565.501742898304,6.67731585723454,38.2914195432042));
#87387=CARTESIAN_POINT('Ctrl Pts',(565.568128174205,6.58507480169042,38.3446749414529));
#87388=CARTESIAN_POINT('Ctrl Pts',(565.647587234012,6.51064311812612,38.387648093995));
#87389=CARTESIAN_POINT('Origin',(565.,18.25,31.609927238132));
#87390=CARTESIAN_POINT('',(521.,18.25,31.609927238132));
#87391=CARTESIAN_POINT('',(565.,18.25,31.609927238132));
#87392=CARTESIAN_POINT('Origin',(521.,18.25,31.609927238132));
#87393=CARTESIAN_POINT('Origin',(640.,11.0311453091351,1.33942354064812));
#87394=CARTESIAN_POINT('',(675.,12.0302566897884,1.29727559824433));
#87395=CARTESIAN_POINT('',(675.,11.8,0.7));
#87396=CARTESIAN_POINT('Origin',(675.,11.0311453091351,1.33942354064812));
#87397=CARTESIAN_POINT('',(640.,11.8,0.7));
#87398=CARTESIAN_POINT('',(640.,11.8,0.7));
#87399=CARTESIAN_POINT('',(640.,11.6246344106287,2.14426556639495));
#87400=CARTESIAN_POINT('Origin',(640.,11.0311453091351,1.33942354064812));
#87401=CARTESIAN_POINT('',(675.,11.6246344106287,2.14426556639495));
#87402=CARTESIAN_POINT('',(640.,11.6246344106287,2.14426556639495));
#87403=CARTESIAN_POINT('',(675.,11.991137666043,1.61944974420474));
#87404=CARTESIAN_POINT('Origin',(675.,11.0311453091351,1.33942354064812));
#87405=CARTESIAN_POINT('Ctrl Pts',(675.,11.991137666043,1.61944974420473));
#87406=CARTESIAN_POINT('Ctrl Pts',(674.991906182189,12.0063466422278,1.56730997761014));
#87407=CARTESIAN_POINT('Ctrl Pts',(674.987834493111,12.0173230229604,1.51374916504173));
#87408=CARTESIAN_POINT('Ctrl Pts',(674.987834493111,12.0303853435058,1.40617127676514));
#87409=CARTESIAN_POINT('Ctrl Pts',(674.991906182189,12.0325458578881,1.35154002422067));
#87410=CARTESIAN_POINT('Ctrl Pts',(675.,12.0302566897884,1.29727559824433));
#87411=CARTESIAN_POINT('',(668.,11.8454198043642,1.91990355444644));
#87412=CARTESIAN_POINT('',(668.,11.9606764275243,0.970679862809448));
#87413=CARTESIAN_POINT('Origin',(668.,11.0311453091351,1.33942354064812));
#87414=CARTESIAN_POINT('',(669.6,11.9606764275243,0.970679862809448));
#87415=CARTESIAN_POINT('',(640.,11.9606764275243,0.97067986280945));
#87416=CARTESIAN_POINT('',(669.6,11.8454198043642,1.91990355444644));
#87417=CARTESIAN_POINT('Origin',(669.6,11.0311453091351,1.33942354064812));
#87418=CARTESIAN_POINT('',(640.,11.8454198043642,1.91990355444644));
#87419=CARTESIAN_POINT('Origin',(668.8,0.,0.));
#87420=CARTESIAN_POINT('Origin',(668.,0.,0.));
#87421=CARTESIAN_POINT('Origin',(669.6,0.,0.));
#87422=CARTESIAN_POINT('Origin',(668.,12.,0.));
#87423=CARTESIAN_POINT('Origin',(640.,13.4,0.7));
#87424=CARTESIAN_POINT('',(640.,12.7808450424845,0.7));
#87425=CARTESIAN_POINT('',(640.,12.8809937504837,0.7));
#87426=CARTESIAN_POINT('',(640.,13.15,0.7));
#87427=CARTESIAN_POINT('',(639.994987437107,12.8809937504837,0.7));
#87428=CARTESIAN_POINT('Ctrl Pts',(640.,12.7808450424844,0.7));
#87429=CARTESIAN_POINT('Ctrl Pts',(640.,12.8130328504931,0.7));
#87430=CARTESIAN_POINT('Ctrl Pts',(639.99842431193,12.8467468199585,0.7));
#87431=CARTESIAN_POINT('Ctrl Pts',(639.994987437107,12.8809937504837,0.7));
#87432=CARTESIAN_POINT('',(654.,12.8809937504837,0.7));
#87433=CARTESIAN_POINT('Origin',(675.,0.,0.));
#87434=CARTESIAN_POINT('Origin',(675.,0.,0.));
#87435=CARTESIAN_POINT('',(675.,11.2895924806261,3.50358411079142));
#87436=CARTESIAN_POINT('',(675.,11.3733529631268,3.1637544746923));
#87437=CARTESIAN_POINT('',(675.,11.3702209229272,4.13860799832838));
#87438=CARTESIAN_POINT('Origin',(675.,10.3900552403499,3.94042819436835));
#87439=CARTESIAN_POINT('',(675.,11.2551373071591,4.44205855398094));
#87440=CARTESIAN_POINT('Origin',(675.,0.,0.));
#87441=CARTESIAN_POINT('',(675.,10.7736873231385,4.86391421215922));
#87442=CARTESIAN_POINT('Origin',(675.,10.3900552403499,3.94042819436835));
#87443=CARTESIAN_POINT('',(675.,10.1230748822772,6.10355264807372));
#87444=CARTESIAN_POINT('',(675.,10.2857279924926,5.79364303909509));
#87445=CARTESIAN_POINT('',(675.,10.0493892450969,6.73941954477757));
#87446=CARTESIAN_POINT('Origin',(675.,9.14513292730969,6.31242948430561));
#87447=CARTESIAN_POINT('',(675.,9.86502927874265,7.00651106682565));
#87448=CARTESIAN_POINT('Origin',(675.,0.,0.));
#87449=CARTESIAN_POINT('',(675.,9.29661268918755,7.30088984352161));
#87450=CARTESIAN_POINT('Origin',(675.,9.14513292730969,6.31242948430561));
#87451=CARTESIAN_POINT('',(675.,8.36824096765044,8.34880489096115));
#87452=CARTESIAN_POINT('',(675.,8.60033389803472,8.08682612910127));
#87453=CARTESIAN_POINT('',(675.,8.14452359238525,8.9485605240776));
#87454=CARTESIAN_POINT('Origin',(675.,7.36872872973994,8.31757531736262));
#87455=CARTESIAN_POINT('',(675.,7.9016016065681,9.16377062409794));
#87456=CARTESIAN_POINT('Origin',(675.,0.,0.));
#87457=CARTESIAN_POINT('',(675.,7.2792527175532,9.31356429483334));
#87458=CARTESIAN_POINT('Origin',(675.,7.36872872973994,8.31757531736262));
#87459=CARTESIAN_POINT('',(675.,6.12707530530208,10.108854940257));
#87460=CARTESIAN_POINT('',(675.,6.41511965836486,9.91003227890105));
#87461=CARTESIAN_POINT('',(675.,5.76632783262284,10.6376436924123));
#87462=CARTESIAN_POINT('Origin',(675.,5.16408080263683,9.83933390613066));
#87463=CARTESIAN_POINT('',(675.,5.47896157017303,10.7884651416486));
#87464=CARTESIAN_POINT('Origin',(675.,0.,0.));
#87465=CARTESIAN_POINT('',(675.,4.83884903698171,10.7849682427581));
#87466=CARTESIAN_POINT('Origin',(675.,5.16408080263683,9.83933390613066));
#87467=CARTESIAN_POINT('',(675.,3.52982629722213,11.2814150846177));
#87468=CARTESIAN_POINT('',(675.,3.85708198216203,11.1573033741528));
#87469=CARTESIAN_POINT('',(675.,3.05301405897726,11.7085056756055));
#87470=CARTESIAN_POINT('Origin',(675.,2.65931526995444,10.7892661727979));
#87471=CARTESIAN_POINT('',(675.,2.7379042025345,11.7861732796419));
#87472=CARTESIAN_POINT('Origin',(675.,0.,0.));
#87473=CARTESIAN_POINT('',(675.,2.11722903888145,11.6295890381783));
#87474=CARTESIAN_POINT('Origin',(675.,2.65931526995444,10.7892661727979));
#87475=CARTESIAN_POINT('',(675.,0.727436615144177,11.7983403905358));
#87476=CARTESIAN_POINT('',(675.,1.0748847210785,11.7561525524464));
#87477=CARTESIAN_POINT('',(675.,0.162270205478485,12.0989118676191));
#87478=CARTESIAN_POINT('Origin',(675.,3.12891701579224E-15,11.112165506889));
#87479=CARTESIAN_POINT('',(675.,-0.162270205478478,12.0989118676191));
#87480=CARTESIAN_POINT('Origin',(675.,0.,0.));
#87481=CARTESIAN_POINT('',(675.,-0.727436615144172,11.7983403905358));
#87482=CARTESIAN_POINT('Origin',(675.,3.12891701579224E-15,11.112165506889));
#87483=CARTESIAN_POINT('',(675.,-2.11722903888145,11.6295890381783));
#87484=CARTESIAN_POINT('',(675.,-1.76978093294713,11.6717768762677));
#87485=CARTESIAN_POINT('',(675.,-2.7379042025345,11.7861732796419));
#87486=CARTESIAN_POINT('Origin',(675.,-2.65931526995444,10.7892661727979));
#87487=CARTESIAN_POINT('',(675.,-3.05301405897725,11.7085056756055));
#87488=CARTESIAN_POINT('Origin',(675.,0.,0.));
#87489=CARTESIAN_POINT('',(675.,-3.52982629722213,11.2814150846177));
#87490=CARTESIAN_POINT('Origin',(675.,-2.65931526995444,10.7892661727979));
#87491=CARTESIAN_POINT('',(675.,-4.83884903698171,10.7849682427581));
#87492=CARTESIAN_POINT('',(675.,-4.51159335204181,10.909079953223));
#87493=CARTESIAN_POINT('',(675.,-5.47896157017303,10.7884651416486));
#87494=CARTESIAN_POINT('Origin',(675.,-5.16408080263683,9.83933390613067));
#87495=CARTESIAN_POINT('',(675.,-5.76632783262284,10.6376436924123));
#87496=CARTESIAN_POINT('Origin',(675.,0.,0.));
#87497=CARTESIAN_POINT('',(675.,-6.12707530530208,10.108854940257));
#87498=CARTESIAN_POINT('Origin',(675.,-5.16408080263683,9.83933390613067));
#87499=CARTESIAN_POINT('',(675.,-7.2792527175532,9.31356429483334));
#87500=CARTESIAN_POINT('',(675.,-6.99120836449042,9.51238695618924));
#87501=CARTESIAN_POINT('',(675.,-7.90160160656809,9.16377062409795));
#87502=CARTESIAN_POINT('Origin',(675.,-7.36872872973994,8.31757531736262));
#87503=CARTESIAN_POINT('',(675.,-8.14452359238525,8.9485605240776));
#87504=CARTESIAN_POINT('Origin',(675.,0.,0.));
#87505=CARTESIAN_POINT('',(675.,-8.36824096765043,8.34880489096116));
#87506=CARTESIAN_POINT('Origin',(675.,-7.36872872973994,8.31757531736262));
#87507=CARTESIAN_POINT('',(675.,-9.29661268918755,7.30088984352162));
#87508=CARTESIAN_POINT('',(675.,-9.06451975880327,7.5628686053815));
#87509=CARTESIAN_POINT('',(675.,-9.86502927874264,7.00651106682565));
#87510=CARTESIAN_POINT('Origin',(675.,-9.14513292730969,6.31242948430562));
#87511=CARTESIAN_POINT('',(675.,-10.0493892450969,6.73941954477757));
#87512=CARTESIAN_POINT('Origin',(675.,0.,0.));
#87513=CARTESIAN_POINT('',(675.,-10.1230748822772,6.10355264807372));
#87514=CARTESIAN_POINT('Origin',(675.,-9.14513292730969,6.31242948430562));
#87515=CARTESIAN_POINT('',(675.,-10.7736873231385,4.86391421215922));
#87516=CARTESIAN_POINT('',(675.,-10.6110342129232,5.17382382113785));
#87517=CARTESIAN_POINT('',(675.,-11.2551373071591,4.44205855398094));
#87518=CARTESIAN_POINT('Origin',(675.,-10.3900552403499,3.94042819436835));
#87519=CARTESIAN_POINT('',(675.,-11.3702209229272,4.13860799832838));
#87520=CARTESIAN_POINT('Origin',(675.,0.,0.));
#87521=CARTESIAN_POINT('',(675.,-11.2895924806261,3.50358411079142));
#87522=CARTESIAN_POINT('Origin',(675.,-10.3900552403499,3.94042819436835));
#87523=CARTESIAN_POINT('',(675.,-11.6246344106287,2.14426556639495));
#87524=CARTESIAN_POINT('',(675.,-11.5408739281281,2.48409520249407));
#87525=CARTESIAN_POINT('',(675.,-11.991137666043,1.61944974420474));
#87526=CARTESIAN_POINT('Origin',(675.,-11.0311453091351,1.33942354064812));
#87527=CARTESIAN_POINT('',(675.,-12.0302566897884,1.29727559824434));
#87528=CARTESIAN_POINT('Origin',(675.,0.,0.));
#87529=CARTESIAN_POINT('',(675.,-11.8,0.700000000000001));
#87530=CARTESIAN_POINT('Origin',(675.,-11.0311453091351,1.33942354064812));
#87531=CARTESIAN_POINT('',(675.,-11.8,-0.699999999999999));
#87532=CARTESIAN_POINT('',(675.,-11.8,-0.349999999999999));
#87533=CARTESIAN_POINT('',(675.,-12.0302566897884,-1.29727559824433));
#87534=CARTESIAN_POINT('Origin',(675.,-11.0311453091351,-1.33942354064811));
#87535=CARTESIAN_POINT('',(675.,-11.991137666043,-1.61944974420474));
#87536=CARTESIAN_POINT('Origin',(675.,0.,0.));
#87537=CARTESIAN_POINT('',(675.,-11.6246344106287,-2.14426556639494));
#87538=CARTESIAN_POINT('Origin',(675.,-11.0311453091351,-1.33942354064811));
#87539=CARTESIAN_POINT('',(675.,-11.2895924806261,-3.50358411079141));
#87540=CARTESIAN_POINT('',(675.,-11.3733529631268,-3.1637544746923));
#87541=CARTESIAN_POINT('',(675.,-11.3702209229272,-4.13860799832838));
#87542=CARTESIAN_POINT('Origin',(675.,-10.3900552403499,-3.94042819436835));
#87543=CARTESIAN_POINT('',(675.,-11.2551373071591,-4.44205855398094));
#87544=CARTESIAN_POINT('Origin',(675.,0.,0.));
#87545=CARTESIAN_POINT('',(675.,-10.7736873231385,-4.86391421215922));
#87546=CARTESIAN_POINT('Origin',(675.,-10.3900552403499,-3.94042819436835));
#87547=CARTESIAN_POINT('',(675.,-10.1230748822772,-6.10355264807372));
#87548=CARTESIAN_POINT('',(675.,-10.2857279924926,-5.79364303909509));
#87549=CARTESIAN_POINT('',(675.,-10.0493892450969,-6.73941954477757));
#87550=CARTESIAN_POINT('Origin',(675.,-9.14513292730969,-6.31242948430561));
#87551=CARTESIAN_POINT('',(675.,-9.86502927874265,-7.00651106682565));
#87552=CARTESIAN_POINT('Origin',(675.,0.,0.));
#87553=CARTESIAN_POINT('',(675.,-9.29661268918755,-7.30088984352161));
#87554=CARTESIAN_POINT('Origin',(675.,-9.14513292730969,-6.31242948430561));
#87555=CARTESIAN_POINT('',(675.,-8.36824096765044,-8.34880489096115));
#87556=CARTESIAN_POINT('',(675.,-8.60033389803472,-8.08682612910127));
#87557=CARTESIAN_POINT('',(675.,-8.14452359238525,-8.9485605240776));
#87558=CARTESIAN_POINT('Origin',(675.,-7.36872872973994,-8.31757531736262));
#87559=CARTESIAN_POINT('',(675.,-7.9016016065681,-9.16377062409794));
#87560=CARTESIAN_POINT('Origin',(675.,0.,0.));
#87561=CARTESIAN_POINT('',(675.,-7.2792527175532,-9.31356429483334));
#87562=CARTESIAN_POINT('Origin',(675.,-7.36872872973994,-8.31757531736262));
#87563=CARTESIAN_POINT('',(675.,-6.12707530530208,-10.108854940257));
#87564=CARTESIAN_POINT('',(675.,-6.41511965836486,-9.91003227890105));
#87565=CARTESIAN_POINT('',(675.,-5.76632783262284,-10.6376436924123));
#87566=CARTESIAN_POINT('Origin',(675.,-5.16408080263683,-9.83933390613066));
#87567=CARTESIAN_POINT('',(675.,-5.47896157017303,-10.7884651416486));
#87568=CARTESIAN_POINT('Origin',(675.,0.,0.));
#87569=CARTESIAN_POINT('',(675.,-4.83884903698172,-10.7849682427581));
#87570=CARTESIAN_POINT('Origin',(675.,-5.16408080263683,-9.83933390613066));
#87571=CARTESIAN_POINT('',(675.,-3.52982629722213,-11.2814150846177));
#87572=CARTESIAN_POINT('',(675.,-3.85708198216203,-11.1573033741528));
#87573=CARTESIAN_POINT('',(675.,-3.05301405897726,-11.7085056756055));
#87574=CARTESIAN_POINT('Origin',(675.,-2.65931526995444,-10.7892661727979));
#87575=CARTESIAN_POINT('',(675.,-2.73790420253451,-11.7861732796419));
#87576=CARTESIAN_POINT('Origin',(675.,0.,0.));
#87577=CARTESIAN_POINT('',(675.,-2.11722903888146,-11.6295890381783));
#87578=CARTESIAN_POINT('Origin',(675.,-2.65931526995444,-10.7892661727979));
#87579=CARTESIAN_POINT('',(675.,-0.72743661514418,-11.7983403905358));
#87580=CARTESIAN_POINT('',(675.,-1.0748847210785,-11.7561525524464));
#87581=CARTESIAN_POINT('',(675.,-0.162270205478491,-12.0989118676191));
#87582=CARTESIAN_POINT('Origin',(675.,-8.40247638276174E-15,-11.112165506889));
#87583=CARTESIAN_POINT('',(675.,0.162270205478472,-12.0989118676191));
#87584=CARTESIAN_POINT('Origin',(675.,0.,0.));
#87585=CARTESIAN_POINT('',(675.,0.727436615144166,-11.7983403905358));
#87586=CARTESIAN_POINT('Origin',(675.,-8.40247638276174E-15,-11.112165506889));
#87587=CARTESIAN_POINT('',(675.,2.11722903888144,-11.6295890381783));
#87588=CARTESIAN_POINT('',(675.,1.76978093294712,-11.6717768762677));
#87589=CARTESIAN_POINT('',(675.,2.7379042025345,-11.7861732796419));
#87590=CARTESIAN_POINT('Origin',(675.,2.65931526995443,-10.7892661727979));
#87591=CARTESIAN_POINT('',(675.,3.05301405897725,-11.7085056756055));
#87592=CARTESIAN_POINT('Origin',(675.,0.,0.));
#87593=CARTESIAN_POINT('',(675.,3.52982629722213,-11.2814150846177));
#87594=CARTESIAN_POINT('Origin',(675.,2.65931526995443,-10.7892661727979));
#87595=CARTESIAN_POINT('',(675.,4.83884903698171,-10.7849682427581));
#87596=CARTESIAN_POINT('',(675.,4.51159335204181,-10.909079953223));
#87597=CARTESIAN_POINT('',(675.,5.47896157017303,-10.7884651416486));
#87598=CARTESIAN_POINT('Origin',(675.,5.16408080263683,-9.83933390613066));
#87599=CARTESIAN_POINT('',(675.,5.76632783262284,-10.6376436924123));
#87600=CARTESIAN_POINT('Origin',(675.,0.,0.));
#87601=CARTESIAN_POINT('',(675.,6.12707530530208,-10.108854940257));
#87602=CARTESIAN_POINT('Origin',(675.,5.16408080263683,-9.83933390613066));
#87603=CARTESIAN_POINT('',(675.,7.2792527175532,-9.31356429483334));
#87604=CARTESIAN_POINT('',(675.,6.99120836449042,-9.51238695618924));
#87605=CARTESIAN_POINT('',(675.,7.90160160656809,-9.16377062409795));
#87606=CARTESIAN_POINT('Origin',(675.,7.36872872973994,-8.31757531736262));
#87607=CARTESIAN_POINT('',(675.,8.14452359238525,-8.94856052407761));
#87608=CARTESIAN_POINT('Origin',(675.,0.,0.));
#87609=CARTESIAN_POINT('',(675.,8.36824096765043,-8.34880489096116));
#87610=CARTESIAN_POINT('Origin',(675.,7.36872872973994,-8.31757531736262));
#87611=CARTESIAN_POINT('',(675.,9.29661268918755,-7.30088984352162));
#87612=CARTESIAN_POINT('',(675.,9.06451975880327,-7.5628686053815));
#87613=CARTESIAN_POINT('',(675.,9.86502927874264,-7.00651106682566));
#87614=CARTESIAN_POINT('Origin',(675.,9.14513292730969,-6.31242948430562));
#87615=CARTESIAN_POINT('',(675.,10.0493892450969,-6.73941954477758));
#87616=CARTESIAN_POINT('Origin',(675.,0.,0.));
#87617=CARTESIAN_POINT('',(675.,10.1230748822772,-6.10355264807372));
#87618=CARTESIAN_POINT('Origin',(675.,9.14513292730969,-6.31242948430562));
#87619=CARTESIAN_POINT('',(675.,10.7736873231385,-4.86391421215923));
#87620=CARTESIAN_POINT('',(675.,10.6110342129232,-5.17382382113785));
#87621=CARTESIAN_POINT('',(675.,11.2551373071591,-4.44205855398095));
#87622=CARTESIAN_POINT('Origin',(675.,10.3900552403499,-3.94042819436836));
#87623=CARTESIAN_POINT('',(675.,11.3702209229272,-4.13860799832839));
#87624=CARTESIAN_POINT('Origin',(675.,0.,0.));
#87625=CARTESIAN_POINT('',(675.,11.2895924806261,-3.50358411079143));
#87626=CARTESIAN_POINT('Origin',(675.,10.3900552403499,-3.94042819436836));
#87627=CARTESIAN_POINT('',(675.,11.6246344106287,-2.14426556639496));
#87628=CARTESIAN_POINT('',(675.,11.5408739281281,-2.48409520249407));
#87629=CARTESIAN_POINT('',(675.,11.991137666043,-1.61944974420488));
#87630=CARTESIAN_POINT('Origin',(675.,11.0311453091351,-1.33942354064812));
#87631=CARTESIAN_POINT('',(675.,12.0302566897885,-1.2972755982442));
#87632=CARTESIAN_POINT('Origin',(675.,0.,0.));
#87633=CARTESIAN_POINT('',(675.,11.8,-0.7));
#87634=CARTESIAN_POINT('Origin',(675.,11.0311453091351,-1.33942354064812));
#87635=CARTESIAN_POINT('',(675.,11.8,0.35));
#87636=CARTESIAN_POINT('Origin',(674.6,0.,0.));
#87637=CARTESIAN_POINT('Origin',(640.,11.8425123594527,1.16828978263508));
#87638=CARTESIAN_POINT('',(640.,12.8376814652891,1.26646539462122));
#87639=CARTESIAN_POINT('',(640.,12.6858443317755,1.70568273426187));
#87640=CARTESIAN_POINT('Origin',(640.,11.8425123594527,1.16828978263508));
#87641=CARTESIAN_POINT('',(639.994987437107,12.8376814652891,1.26646539462122));
#87642=CARTESIAN_POINT('',(640.,12.8376814652891,1.26646539462122));
#87643=CARTESIAN_POINT('Ctrl Pts',(640.,12.6858443317753,1.70568273426216));
#87644=CARTESIAN_POINT('Ctrl Pts',(640.,12.7039865654686,1.67721208596548));
#87645=CARTESIAN_POINT('Ctrl Pts',(639.999699519233,12.7208347539922,1.64759178154739));
#87646=CARTESIAN_POINT('Ctrl Pts',(639.997691867076,12.7911973493947,1.50740766279947));
#87647=CARTESIAN_POINT('Ctrl Pts',(639.994987437107,12.8256145545127,1.38878311247967));
#87648=CARTESIAN_POINT('Ctrl Pts',(639.994987437107,12.8376814652891,1.26646539462123));
#87649=CARTESIAN_POINT('Origin',(669.6,12.9,0.));
#87650=CARTESIAN_POINT('Origin',(640.,10.3900552403499,3.94042819436835));
#87651=CARTESIAN_POINT('',(640.,10.7736873231385,4.86391421215922));
#87652=CARTESIAN_POINT('',(640.,11.2895924806261,3.50358411079142));
#87653=CARTESIAN_POINT('Origin',(640.,10.3900552403499,3.94042819436835));
#87654=CARTESIAN_POINT('',(640.,10.7736873231385,4.86391421215922));
#87655=CARTESIAN_POINT('Ctrl Pts',(675.,11.2551373071591,4.44205855398094));
#87656=CARTESIAN_POINT('Ctrl Pts',(674.991906182189,11.2823822010156,4.39507362048221));
#87657=CARTESIAN_POINT('Ctrl Pts',(674.987834493111,11.3058575695124,4.34569600763073));
#87658=CARTESIAN_POINT('Ctrl Pts',(674.987834493111,11.3442853965581,4.24437015519104));
#87659=CARTESIAN_POINT('Ctrl Pts',(674.991906182189,11.3594572448126,4.19184343249186));
#87660=CARTESIAN_POINT('Ctrl Pts',(675.,11.3702209229272,4.13860799832838));
#87661=CARTESIAN_POINT('',(640.,11.2895924806261,3.50358411079142));
#87662=CARTESIAN_POINT('',(668.,11.0417504385235,4.69890915568338));
#87663=CARTESIAN_POINT('',(668.,11.3808220120066,3.80485089471659));
#87664=CARTESIAN_POINT('Origin',(668.,10.3900552403499,3.94042819436835));
#87665=CARTESIAN_POINT('',(669.6,11.3808220120066,3.80485089471659));
#87666=CARTESIAN_POINT('',(640.,11.3808220120066,3.8048508947166));
#87667=CARTESIAN_POINT('',(669.6,11.0417504385235,4.69890915568338));
#87668=CARTESIAN_POINT('Origin',(669.6,10.3900552403499,3.94042819436835));
#87669=CARTESIAN_POINT('',(640.,11.0417504385235,4.69890915568338));
#87670=CARTESIAN_POINT('Origin',(668.8,0.,0.));
#87671=CARTESIAN_POINT('Origin',(668.,0.,0.));
#87672=CARTESIAN_POINT('Origin',(669.6,0.,0.));
#87673=CARTESIAN_POINT('Origin',(668.,12.,0.));
#87674=CARTESIAN_POINT('Origin',(674.6,0.,0.));
#87675=CARTESIAN_POINT('Origin',(669.6,12.9,0.));
#87676=CARTESIAN_POINT('Origin',(640.,9.14513292730969,6.31242948430561));
#87677=CARTESIAN_POINT('',(640.,9.29661268918755,7.30088984352161));
#87678=CARTESIAN_POINT('',(640.,10.1230748822772,6.10355264807372));
#87679=CARTESIAN_POINT('Origin',(640.,9.14513292730969,6.31242948430561));
#87680=CARTESIAN_POINT('',(640.,9.29661268918755,7.30088984352161));
#87681=CARTESIAN_POINT('Ctrl Pts',(675.,9.86502927874265,7.00651106682565));
#87682=CARTESIAN_POINT('Ctrl Pts',(674.991906182189,9.90272671607098,6.96741155997444));
#87683=CARTESIAN_POINT('Ctrl Pts',(674.987834493111,9.93733676924454,6.92508679421849));
#87684=CARTESIAN_POINT('Ctrl Pts',(674.987834493111,9.99889681716215,6.83590166785504));
#87685=CARTESIAN_POINT('Ctrl Pts',(674.991906182189,10.0261982666157,6.78853213719756));
#87686=CARTESIAN_POINT('Ctrl Pts',(675.,10.0493892450969,6.73941954477757));
#87687=CARTESIAN_POINT('',(640.,10.1230748822772,6.10355264807372));
#87688=CARTESIAN_POINT('',(668.,9.5963746723257,7.20483123663183));
#87689=CARTESIAN_POINT('',(668.,10.1395555887559,6.41789782269309));
#87690=CARTESIAN_POINT('Origin',(668.,9.14513292730969,6.31242948430561));
#87691=CARTESIAN_POINT('',(669.6,10.1395555887559,6.41789782269309));
#87692=CARTESIAN_POINT('',(640.,10.1395555887559,6.4178978226931));
#87693=CARTESIAN_POINT('',(669.6,9.5963746723257,7.20483123663183));
#87694=CARTESIAN_POINT('Origin',(669.6,9.14513292730969,6.31242948430561));
#87695=CARTESIAN_POINT('',(640.,9.59637467232571,7.20483123663183));
#87696=CARTESIAN_POINT('Origin',(668.8,0.,0.));
#87697=CARTESIAN_POINT('Origin',(668.,0.,0.));
#87698=CARTESIAN_POINT('Origin',(669.6,0.,0.));
#87699=CARTESIAN_POINT('Origin',(668.,12.,0.));
#87700=CARTESIAN_POINT('Origin',(674.6,0.,0.));
#87701=CARTESIAN_POINT('Origin',(669.6,12.9,0.));
#87702=CARTESIAN_POINT('Origin',(640.,7.36872872973994,8.31757531736262));
#87703=CARTESIAN_POINT('',(640.,7.2792527175532,9.31356429483334));
#87704=CARTESIAN_POINT('',(640.,8.36824096765044,8.34880489096115));
#87705=CARTESIAN_POINT('Origin',(640.,7.36872872973994,8.31757531736262));
#87706=CARTESIAN_POINT('',(640.,7.2792527175532,9.31356429483334));
#87707=CARTESIAN_POINT('Ctrl Pts',(675.,7.9016016065681,9.16377062409794));
#87708=CARTESIAN_POINT('Ctrl Pts',(674.991906182189,7.94756074933538,9.13482886511155));
#87709=CARTESIAN_POINT('Ctrl Pts',(674.987834493111,7.99129407669763,9.10201670799259));
#87710=CARTESIAN_POINT('Ctrl Pts',(674.987834493111,8.07240869926383,9.03015542307487));
#87711=CARTESIAN_POINT('Ctrl Pts',(674.991906182189,8.11025308891089,8.99069602939966));
#87712=CARTESIAN_POINT('Ctrl Pts',(675.,8.14452359238525,8.9485605240776));
#87713=CARTESIAN_POINT('',(640.,8.36824096765044,8.34880489096115));
#87714=CARTESIAN_POINT('',(668.,7.59329249157496,9.29203471460322));
#87715=CARTESIAN_POINT('',(668.,8.30901505047168,8.65795985732407));
#87716=CARTESIAN_POINT('Origin',(668.,7.36872872973994,8.31757531736262));
#87717=CARTESIAN_POINT('',(669.6,8.30901505047168,8.65795985732407));
#87718=CARTESIAN_POINT('',(640.,8.30901505047168,8.65795985732407));
#87719=CARTESIAN_POINT('',(669.6,7.59329249157496,9.29203471460322));
#87720=CARTESIAN_POINT('Origin',(669.6,7.36872872973994,8.31757531736262));
#87721=CARTESIAN_POINT('',(640.,7.59329249157496,9.29203471460322));
#87722=CARTESIAN_POINT('Origin',(668.8,0.,0.));
#87723=CARTESIAN_POINT('Origin',(668.,0.,0.));
#87724=CARTESIAN_POINT('Origin',(669.6,0.,0.));
#87725=CARTESIAN_POINT('Origin',(668.,12.,0.));
#87726=CARTESIAN_POINT('Origin',(674.6,0.,0.));
#87727=CARTESIAN_POINT('Origin',(669.6,12.9,0.));
#87728=CARTESIAN_POINT('Origin',(640.,5.16408080263683,9.83933390613066));
#87729=CARTESIAN_POINT('',(640.,4.83884903698171,10.7849682427581));
#87730=CARTESIAN_POINT('',(640.,6.12707530530208,10.108854940257));
#87731=CARTESIAN_POINT('Origin',(640.,5.16408080263683,9.83933390613066));
#87732=CARTESIAN_POINT('',(640.,4.83884903698171,10.7849682427581));
#87733=CARTESIAN_POINT('Ctrl Pts',(675.,5.47896157017303,10.7884651416486));
#87734=CARTESIAN_POINT('Ctrl Pts',(674.991906182189,5.53051144005632,10.7713631203603));
#87735=CARTESIAN_POINT('Ctrl Pts',(674.987834493111,5.58082641958515,10.7499704951827));
#87736=CARTESIAN_POINT('Ctrl Pts',(674.987834493111,5.67678152977602,10.699609368385));
#87737=CARTESIAN_POINT('Ctrl Pts',(674.991906182189,5.72296948124909,10.6703533482234));
#87738=CARTESIAN_POINT('Ctrl Pts',(675.,5.76632783262284,10.6376436924123));
#87739=CARTESIAN_POINT('',(640.,6.12707530530208,10.108854940257));
#87740=CARTESIAN_POINT('',(668.,5.14891575170907,10.8392189101338));
#87741=CARTESIAN_POINT('',(668.,5.99558475949487,10.394852735451));
#87742=CARTESIAN_POINT('Origin',(668.,5.16408080263683,9.83933390613066));
#87743=CARTESIAN_POINT('',(669.6,5.99558475949487,10.394852735451));
#87744=CARTESIAN_POINT('',(640.,5.99558475949487,10.394852735451));
#87745=CARTESIAN_POINT('',(669.6,5.14891575170907,10.8392189101338));
#87746=CARTESIAN_POINT('Origin',(669.6,5.16408080263683,9.83933390613066));
#87747=CARTESIAN_POINT('',(640.,5.14891575170907,10.8392189101338));
#87748=CARTESIAN_POINT('Origin',(668.8,0.,0.));
#87749=CARTESIAN_POINT('Origin',(668.,0.,0.));
#87750=CARTESIAN_POINT('Origin',(669.6,0.,0.));
#87751=CARTESIAN_POINT('Origin',(668.,12.,0.));
#87752=CARTESIAN_POINT('Origin',(674.6,0.,0.));
#87753=CARTESIAN_POINT('Origin',(669.6,12.9,0.));
#87754=CARTESIAN_POINT('Origin',(640.,2.65931526995444,10.7892661727979));
#87755=CARTESIAN_POINT('',(640.,2.11722903888145,11.6295890381783));
#87756=CARTESIAN_POINT('',(640.,3.52982629722213,11.2814150846177));
#87757=CARTESIAN_POINT('Origin',(640.,2.65931526995444,10.7892661727979));
#87758=CARTESIAN_POINT('',(640.,2.11722903888145,11.6295890381783));
#87759=CARTESIAN_POINT('Ctrl Pts',(675.,2.7379042025345,11.7861732796419));
#87760=CARTESIAN_POINT('Ctrl Pts',(674.991906182189,2.79204890847233,11.7819049033656));
#87761=CARTESIAN_POINT('Ctrl Pts',(674.987834493111,2.84602141644503,11.7731750717457));
#87762=CARTESIAN_POINT('Ctrl Pts',(674.987834493111,2.95124045203896,11.7472409087023));
#87763=CARTESIAN_POINT('Ctrl Pts',(674.991906182189,3.00308768948478,11.7298885156048));
#87764=CARTESIAN_POINT('Ctrl Pts',(675.,3.05301405897726,11.7085056756055));
#87765=CARTESIAN_POINT('',(640.,3.52982629722213,11.2814150846177));
#87766=CARTESIAN_POINT('',(668.,2.4053027439011,11.7564671015651));
#87767=CARTESIAN_POINT('',(668.,3.3337128753601,11.5276345563458));
#87768=CARTESIAN_POINT('Origin',(668.,2.65931526995444,10.7892661727979));
#87769=CARTESIAN_POINT('',(669.6,3.3337128753601,11.5276345563458));
#87770=CARTESIAN_POINT('',(640.,3.3337128753601,11.5276345563458));
#87771=CARTESIAN_POINT('',(669.6,2.4053027439011,11.7564671015651));
#87772=CARTESIAN_POINT('Origin',(669.6,2.65931526995444,10.7892661727979));
#87773=CARTESIAN_POINT('',(640.,2.40530274390111,11.7564671015651));
#87774=CARTESIAN_POINT('Origin',(668.8,0.,0.));
#87775=CARTESIAN_POINT('Origin',(668.,0.,0.));
#87776=CARTESIAN_POINT('Origin',(669.6,0.,0.));
#87777=CARTESIAN_POINT('Origin',(668.,12.,0.));
#87778=CARTESIAN_POINT('Origin',(674.6,0.,0.));
#87779=CARTESIAN_POINT('Origin',(669.6,12.9,0.));
#87780=CARTESIAN_POINT('Origin',(640.,3.12891701579224E-15,11.112165506889));
#87781=CARTESIAN_POINT('',(640.,-0.727436615144172,11.7983403905358));
#87782=CARTESIAN_POINT('',(640.,0.727436615144177,11.7983403905358));
#87783=CARTESIAN_POINT('Origin',(640.,3.12891701579224E-15,11.112165506889));
#87784=CARTESIAN_POINT('',(640.,-0.727436615144172,11.7983403905358));
#87785=CARTESIAN_POINT('Ctrl Pts',(675.,-0.162270205478478,12.0989118676191));
#87786=CARTESIAN_POINT('Ctrl Pts',(674.991906182189,-0.108677356987216,
12.1077251988691));
#87787=CARTESIAN_POINT('Ctrl Pts',(674.987834493111,-0.0541840065519403,
12.112165506889));
#87788=CARTESIAN_POINT('Ctrl Pts',(674.987834493111,0.0541840065519463,
12.112165506889));
#87789=CARTESIAN_POINT('Ctrl Pts',(674.991906182189,0.108677356987222,12.1077251988691));
#87790=CARTESIAN_POINT('Ctrl Pts',(675.,0.162270205478485,12.0989118676191));
#87791=CARTESIAN_POINT('',(640.,0.727436615144177,11.7983403905358));
#87792=CARTESIAN_POINT('',(668.,-0.478097716462656,11.9904721580726));
#87793=CARTESIAN_POINT('',(668.,0.478097716462662,11.9904721580726));
#87794=CARTESIAN_POINT('Origin',(668.,3.12891701579224E-15,11.112165506889));
#87795=CARTESIAN_POINT('',(669.6,0.478097716462662,11.9904721580726));
#87796=CARTESIAN_POINT('',(640.,0.47809771646266,11.9904721580726));
#87797=CARTESIAN_POINT('',(669.6,-0.478097716462656,11.9904721580726));
#87798=CARTESIAN_POINT('Origin',(669.6,3.12891701579224E-15,11.112165506889));
#87799=CARTESIAN_POINT('',(640.,-0.478097716462654,11.9904721580726));
#87800=CARTESIAN_POINT('Origin',(668.8,0.,0.));
#87801=CARTESIAN_POINT('Origin',(668.,0.,0.));
#87802=CARTESIAN_POINT('Origin',(669.6,0.,0.));
#87803=CARTESIAN_POINT('Origin',(668.,12.,0.));
#87804=CARTESIAN_POINT('Origin',(674.6,0.,0.));
#87805=CARTESIAN_POINT('Origin',(669.6,12.9,0.));
#87806=CARTESIAN_POINT('Origin',(640.,-2.65931526995444,10.7892661727979));
#87807=CARTESIAN_POINT('',(640.,-3.52982629722213,11.2814150846177));
#87808=CARTESIAN_POINT('',(640.,-2.11722903888145,11.6295890381783));
#87809=CARTESIAN_POINT('Origin',(640.,-2.65931526995444,10.7892661727979));
#87810=CARTESIAN_POINT('',(640.,-3.52982629722213,11.2814150846177));
#87811=CARTESIAN_POINT('Ctrl Pts',(675.,-3.05301405897725,11.7085056756055));
#87812=CARTESIAN_POINT('Ctrl Pts',(674.991906182189,-3.00308768948475,11.7298885156048));
#87813=CARTESIAN_POINT('Ctrl Pts',(674.987834493111,-2.95124045203896,11.7472409087023));
#87814=CARTESIAN_POINT('Ctrl Pts',(674.987834493111,-2.84602141644506,11.7731750717457));
#87815=CARTESIAN_POINT('Ctrl Pts',(674.991906182189,-2.79204890847233,11.7819049033656));
#87816=CARTESIAN_POINT('Ctrl Pts',(675.,-2.73790420253451,11.7861732796419));
#87817=CARTESIAN_POINT('',(640.,-2.11722903888145,11.6295890381783));
#87818=CARTESIAN_POINT('',(668.,-3.3337128753601,11.5276345563458));
#87819=CARTESIAN_POINT('',(668.,-2.4053027439011,11.7564671015651));
#87820=CARTESIAN_POINT('Origin',(668.,-2.65931526995444,10.7892661727979));
#87821=CARTESIAN_POINT('',(669.6,-2.4053027439011,11.7564671015651));
#87822=CARTESIAN_POINT('',(640.,-2.4053027439011,11.7564671015651));
#87823=CARTESIAN_POINT('',(669.6,-3.3337128753601,11.5276345563458));
#87824=CARTESIAN_POINT('Origin',(669.6,-2.65931526995444,10.7892661727979));
#87825=CARTESIAN_POINT('',(640.,-3.3337128753601,11.5276345563458));
#87826=CARTESIAN_POINT('Origin',(668.8,0.,0.));
#87827=CARTESIAN_POINT('Origin',(668.,0.,0.));
#87828=CARTESIAN_POINT('Origin',(669.6,0.,0.));
#87829=CARTESIAN_POINT('Origin',(668.,12.,0.));
#87830=CARTESIAN_POINT('Origin',(674.6,0.,0.));
#87831=CARTESIAN_POINT('Origin',(669.6,12.9,0.));
#87832=CARTESIAN_POINT('Origin',(640.,-5.16408080263683,9.83933390613067));
#87833=CARTESIAN_POINT('',(640.,-6.12707530530208,10.108854940257));
#87834=CARTESIAN_POINT('',(640.,-4.83884903698171,10.7849682427581));
#87835=CARTESIAN_POINT('Origin',(640.,-5.16408080263683,9.83933390613067));
#87836=CARTESIAN_POINT('',(640.,-6.12707530530208,10.108854940257));
#87837=CARTESIAN_POINT('Ctrl Pts',(675.,-5.76632783262284,10.6376436924123));
#87838=CARTESIAN_POINT('Ctrl Pts',(674.991906182189,-5.72296948124911,10.6703533482234));
#87839=CARTESIAN_POINT('Ctrl Pts',(674.987834493111,-5.67678152977605,10.699609368385));
#87840=CARTESIAN_POINT('Ctrl Pts',(674.987834493111,-5.58082641958515,10.7499704951827));
#87841=CARTESIAN_POINT('Ctrl Pts',(674.991906182189,-5.53051144005631,10.7713631203603));
#87842=CARTESIAN_POINT('Ctrl Pts',(675.,-5.47896157017303,10.7884651416486));
#87843=CARTESIAN_POINT('',(640.,-4.83884903698171,10.7849682427581));
#87844=CARTESIAN_POINT('',(668.,-5.99558475949487,10.394852735451));
#87845=CARTESIAN_POINT('',(668.,-5.14891575170907,10.8392189101338));
#87846=CARTESIAN_POINT('Origin',(668.,-5.16408080263683,9.83933390613067));
#87847=CARTESIAN_POINT('',(669.6,-5.14891575170907,10.8392189101338));
#87848=CARTESIAN_POINT('',(640.,-5.14891575170907,10.8392189101338));
#87849=CARTESIAN_POINT('',(669.6,-5.99558475949487,10.394852735451));
#87850=CARTESIAN_POINT('Origin',(669.6,-5.16408080263683,9.83933390613067));
#87851=CARTESIAN_POINT('',(640.,-5.99558475949487,10.394852735451));
#87852=CARTESIAN_POINT('Origin',(668.8,0.,0.));
#87853=CARTESIAN_POINT('Origin',(668.,0.,0.));
#87854=CARTESIAN_POINT('Origin',(669.6,0.,0.));
#87855=CARTESIAN_POINT('Origin',(668.,12.,0.));
#87856=CARTESIAN_POINT('Origin',(674.6,0.,0.));
#87857=CARTESIAN_POINT('Origin',(669.6,12.9,0.));
#87858=CARTESIAN_POINT('Origin',(640.,-7.36872872973994,8.31757531736262));
#87859=CARTESIAN_POINT('',(640.,-8.36824096765043,8.34880489096116));
#87860=CARTESIAN_POINT('',(640.,-7.2792527175532,9.31356429483334));
#87861=CARTESIAN_POINT('Origin',(640.,-7.36872872973994,8.31757531736262));
#87862=CARTESIAN_POINT('',(640.,-8.36824096765043,8.34880489096116));
#87863=CARTESIAN_POINT('Ctrl Pts',(675.,-8.14452359238525,8.9485605240776));
#87864=CARTESIAN_POINT('Ctrl Pts',(674.991906182189,-8.11025308891089,8.99069602939965));
#87865=CARTESIAN_POINT('Ctrl Pts',(674.987834493111,-8.07240869926384,9.03015542307486));
#87866=CARTESIAN_POINT('Ctrl Pts',(674.987834493111,-7.99129407669764,9.10201670799257));
#87867=CARTESIAN_POINT('Ctrl Pts',(674.991906182189,-7.94756074933538,9.13482886511155));
#87868=CARTESIAN_POINT('Ctrl Pts',(675.,-7.90160160656809,9.16377062409795));
#87869=CARTESIAN_POINT('',(640.,-7.2792527175532,9.31356429483334));
#87870=CARTESIAN_POINT('',(668.,-8.30901505047168,8.65795985732408));
#87871=CARTESIAN_POINT('',(668.,-7.59329249157495,9.29203471460322));
#87872=CARTESIAN_POINT('Origin',(668.,-7.36872872973994,8.31757531736262));
#87873=CARTESIAN_POINT('',(669.6,-7.59329249157495,9.29203471460322));
#87874=CARTESIAN_POINT('',(640.,-7.59329249157496,9.29203471460322));
#87875=CARTESIAN_POINT('',(669.6,-8.30901505047168,8.65795985732408));
#87876=CARTESIAN_POINT('Origin',(669.6,-7.36872872973994,8.31757531736262));
#87877=CARTESIAN_POINT('',(640.,-8.30901505047167,8.65795985732408));
#87878=CARTESIAN_POINT('Origin',(668.8,0.,0.));
#87879=CARTESIAN_POINT('Origin',(668.,0.,0.));
#87880=CARTESIAN_POINT('Origin',(669.6,0.,0.));
#87881=CARTESIAN_POINT('Origin',(668.,12.,0.));
#87882=CARTESIAN_POINT('Origin',(674.6,0.,0.));
#87883=CARTESIAN_POINT('Origin',(669.6,12.9,0.));
#87884=CARTESIAN_POINT('Origin',(640.,-9.14513292730969,6.31242948430562));
#87885=CARTESIAN_POINT('',(640.,-10.1230748822772,6.10355264807372));
#87886=CARTESIAN_POINT('',(640.,-9.29661268918755,7.30088984352162));
#87887=CARTESIAN_POINT('Origin',(640.,-9.14513292730969,6.31242948430562));
#87888=CARTESIAN_POINT('',(640.,-10.1230748822772,6.10355264807372));
#87889=CARTESIAN_POINT('Ctrl Pts',(675.,-10.0493892450969,6.73941954477758));
#87890=CARTESIAN_POINT('Ctrl Pts',(674.991906182189,-10.0261982666157,6.78853213719755));
#87891=CARTESIAN_POINT('Ctrl Pts',(674.987834493111,-9.99889681716215,6.83590166785506));
#87892=CARTESIAN_POINT('Ctrl Pts',(674.987834493111,-9.93733676924455,6.92508679421847));
#87893=CARTESIAN_POINT('Ctrl Pts',(674.991906182189,-9.90272671607098,6.96741155997444));
#87894=CARTESIAN_POINT('Ctrl Pts',(675.,-9.86502927874264,7.00651106682565));
#87895=CARTESIAN_POINT('',(640.,-9.29661268918755,7.30088984352162));
#87896=CARTESIAN_POINT('',(668.,-10.1395555887559,6.4178978226931));
#87897=CARTESIAN_POINT('',(668.,-9.5963746723257,7.20483123663183));
#87898=CARTESIAN_POINT('Origin',(668.,-9.14513292730969,6.31242948430562));
#87899=CARTESIAN_POINT('',(669.6,-9.5963746723257,7.20483123663183));
#87900=CARTESIAN_POINT('',(640.,-9.5963746723257,7.20483123663184));
#87901=CARTESIAN_POINT('',(669.6,-10.1395555887559,6.4178978226931));
#87902=CARTESIAN_POINT('Origin',(669.6,-9.14513292730969,6.31242948430562));
#87903=CARTESIAN_POINT('',(640.,-10.1395555887559,6.4178978226931));
#87904=CARTESIAN_POINT('Origin',(668.8,0.,0.));
#87905=CARTESIAN_POINT('Origin',(668.,0.,0.));
#87906=CARTESIAN_POINT('Origin',(669.6,0.,0.));
#87907=CARTESIAN_POINT('Origin',(668.,12.,0.));
#87908=CARTESIAN_POINT('Origin',(674.6,0.,0.));
#87909=CARTESIAN_POINT('Origin',(669.6,12.9,0.));
#87910=CARTESIAN_POINT('Origin',(640.,-10.3900552403499,3.94042819436835));
#87911=CARTESIAN_POINT('',(640.,-11.2895924806261,3.50358411079142));
#87912=CARTESIAN_POINT('',(640.,-10.7736873231385,4.86391421215922));
#87913=CARTESIAN_POINT('Origin',(640.,-10.3900552403499,3.94042819436835));
#87914=CARTESIAN_POINT('',(640.,-11.2895924806261,3.50358411079142));
#87915=CARTESIAN_POINT('Ctrl Pts',(675.,-11.3702209229272,4.13860799832839));
#87916=CARTESIAN_POINT('Ctrl Pts',(674.991906182189,-11.3594572448126,4.19184343249189));
#87917=CARTESIAN_POINT('Ctrl Pts',(674.987834493111,-11.3442853965581,4.24437015519105));
#87918=CARTESIAN_POINT('Ctrl Pts',(674.987834493111,-11.3058575695124,4.3456960076307));
#87919=CARTESIAN_POINT('Ctrl Pts',(674.991906182189,-11.2823822010156,4.39507362048219));
#87920=CARTESIAN_POINT('Ctrl Pts',(675.,-11.2551373071591,4.44205855398094));
#87921=CARTESIAN_POINT('',(640.,-10.7736873231385,4.86391421215922));
#87922=CARTESIAN_POINT('',(668.,-11.3808220120066,3.8048508947166));
#87923=CARTESIAN_POINT('',(668.,-11.0417504385235,4.69890915568338));
#87924=CARTESIAN_POINT('Origin',(668.,-10.3900552403499,3.94042819436835));
#87925=CARTESIAN_POINT('',(669.6,-11.0417504385235,4.69890915568338));
#87926=CARTESIAN_POINT('',(640.,-11.0417504385235,4.69890915568338));
#87927=CARTESIAN_POINT('',(669.6,-11.3808220120066,3.8048508947166));
#87928=CARTESIAN_POINT('Origin',(669.6,-10.3900552403499,3.94042819436835));
#87929=CARTESIAN_POINT('',(640.,-11.3808220120066,3.8048508947166));
#87930=CARTESIAN_POINT('Origin',(668.8,0.,0.));
#87931=CARTESIAN_POINT('Origin',(668.,0.,0.));
#87932=CARTESIAN_POINT('Origin',(669.6,0.,0.));
#87933=CARTESIAN_POINT('Origin',(668.,12.,0.));
#87934=CARTESIAN_POINT('Origin',(674.6,0.,0.));
#87935=CARTESIAN_POINT('Origin',(669.6,12.9,0.));
#87936=CARTESIAN_POINT('Origin',(640.,-11.0311453091351,1.33942354064812));
#87937=CARTESIAN_POINT('',(640.,-11.8,0.700000000000001));
#87938=CARTESIAN_POINT('',(640.,-11.6246344106287,2.14426556639495));
#87939=CARTESIAN_POINT('Origin',(640.,-11.0311453091351,1.33942354064812));
#87940=CARTESIAN_POINT('',(640.,-11.8,0.700000000000001));
#87941=CARTESIAN_POINT('Ctrl Pts',(675.,-12.0302566897884,1.29727559824434));
#87942=CARTESIAN_POINT('Ctrl Pts',(674.991906182189,-12.0325458578881,1.35154002422071));
#87943=CARTESIAN_POINT('Ctrl Pts',(674.987834493111,-12.0303853435058,1.40617127676514));
#87944=CARTESIAN_POINT('Ctrl Pts',(674.987834493111,-12.0173230229604,1.51374916504174));
#87945=CARTESIAN_POINT('Ctrl Pts',(674.991906182189,-12.0063466422278,1.56730997761013));
#87946=CARTESIAN_POINT('Ctrl Pts',(675.,-11.991137666043,1.61944974420474));
#87947=CARTESIAN_POINT('',(640.,-11.6246344106287,2.14426556639495));
#87948=CARTESIAN_POINT('',(668.,-11.9606764275243,0.970679862809452));
#87949=CARTESIAN_POINT('',(668.,-11.8454198043642,1.91990355444645));
#87950=CARTESIAN_POINT('Origin',(668.,-11.0311453091351,1.33942354064812));
#87951=CARTESIAN_POINT('',(669.6,-11.8454198043642,1.91990355444645));
#87952=CARTESIAN_POINT('',(640.,-11.8454198043642,1.91990355444645));
#87953=CARTESIAN_POINT('',(669.6,-11.9606764275243,0.970679862809452));
#87954=CARTESIAN_POINT('Origin',(669.6,-11.0311453091351,1.33942354064812));
#87955=CARTESIAN_POINT('',(640.,-11.9606764275243,0.97067986280945));
#87956=CARTESIAN_POINT('Origin',(668.8,0.,0.));
#87957=CARTESIAN_POINT('Origin',(668.,0.,0.));
#87958=CARTESIAN_POINT('Origin',(669.6,0.,0.));
#87959=CARTESIAN_POINT('Origin',(668.,12.,0.));
#87960=CARTESIAN_POINT('Origin',(674.6,0.,0.));
#87961=CARTESIAN_POINT('Origin',(669.6,12.9,0.));
#87962=CARTESIAN_POINT('Origin',(640.,-11.0311453091351,-1.33942354064811));
#87963=CARTESIAN_POINT('',(640.,-11.6246344106287,-2.14426556639494));
#87964=CARTESIAN_POINT('',(640.,-11.8,-0.699999999999999));
#87965=CARTESIAN_POINT('Origin',(640.,-11.0311453091351,-1.33942354064811));
#87966=CARTESIAN_POINT('',(640.,-11.6246344106287,-2.14426556639494));
#87967=CARTESIAN_POINT('Ctrl Pts',(675.,-11.991137666043,-1.61944974420474));
#87968=CARTESIAN_POINT('Ctrl Pts',(674.991906182189,-12.0063466422278,-1.56730997761012));
#87969=CARTESIAN_POINT('Ctrl Pts',(674.987834493111,-12.0173230229604,-1.51374916504174));
#87970=CARTESIAN_POINT('Ctrl Pts',(674.987834493111,-12.0303853435058,-1.40617127676513));
#87971=CARTESIAN_POINT('Ctrl Pts',(674.991906182189,-12.0325458578881,-1.35154002422066));
#87972=CARTESIAN_POINT('Ctrl Pts',(675.,-12.0302566897884,-1.29727559824433));
#87973=CARTESIAN_POINT('',(640.,-11.8,-0.699999999999999));
#87974=CARTESIAN_POINT('',(668.,-11.8454198043642,-1.91990355444644));
#87975=CARTESIAN_POINT('',(668.,-11.9606764275243,-0.970679862809445));
#87976=CARTESIAN_POINT('Origin',(668.,-11.0311453091351,-1.33942354064811));
#87977=CARTESIAN_POINT('',(669.6,-11.9606764275243,-0.970679862809445));
#87978=CARTESIAN_POINT('',(640.,-11.9606764275243,-0.97067986280945));
#87979=CARTESIAN_POINT('',(669.6,-11.8454198043642,-1.91990355444644));
#87980=CARTESIAN_POINT('Origin',(669.6,-11.0311453091351,-1.33942354064811));
#87981=CARTESIAN_POINT('',(640.,-11.8454198043642,-1.91990355444643));
#87982=CARTESIAN_POINT('Origin',(668.8,0.,0.));
#87983=CARTESIAN_POINT('Origin',(668.,0.,0.));
#87984=CARTESIAN_POINT('Origin',(669.6,0.,0.));
#87985=CARTESIAN_POINT('Origin',(668.,12.,0.));
#87986=CARTESIAN_POINT('Origin',(674.6,0.,0.));
#87987=CARTESIAN_POINT('Origin',(669.6,12.9,0.));
#87988=CARTESIAN_POINT('Origin',(640.,-10.3900552403499,-3.94042819436835));
#87989=CARTESIAN_POINT('',(640.,-10.7736873231385,-4.86391421215922));
#87990=CARTESIAN_POINT('',(640.,-11.2895924806261,-3.50358411079141));
#87991=CARTESIAN_POINT('Origin',(640.,-10.3900552403499,-3.94042819436835));
#87992=CARTESIAN_POINT('',(640.,-10.7736873231385,-4.86391421215922));
#87993=CARTESIAN_POINT('Ctrl Pts',(675.,-11.2551373071591,-4.44205855398093));
#87994=CARTESIAN_POINT('Ctrl Pts',(674.991906182189,-11.2823822010156,-4.39507362048221));
#87995=CARTESIAN_POINT('Ctrl Pts',(674.987834493111,-11.3058575695124,-4.3456960076307));
#87996=CARTESIAN_POINT('Ctrl Pts',(674.987834493111,-11.3442853965581,-4.24437015519107));
#87997=CARTESIAN_POINT('Ctrl Pts',(674.991906182189,-11.3594572448126,-4.19184343249187));
#87998=CARTESIAN_POINT('Ctrl Pts',(675.,-11.3702209229272,-4.13860799832838));
#87999=CARTESIAN_POINT('',(640.,-11.2895924806261,-3.50358411079141));
#88000=CARTESIAN_POINT('',(668.,-11.0417504385235,-4.69890915568338));
#88001=CARTESIAN_POINT('',(668.,-11.3808220120066,-3.80485089471659));
#88002=CARTESIAN_POINT('Origin',(668.,-10.3900552403499,-3.94042819436835));
#88003=CARTESIAN_POINT('',(669.6,-11.3808220120066,-3.80485089471659));
#88004=CARTESIAN_POINT('',(640.,-11.3808220120066,-3.80485089471659));
#88005=CARTESIAN_POINT('',(669.6,-11.0417504385235,-4.69890915568338));
#88006=CARTESIAN_POINT('Origin',(669.6,-10.3900552403499,-3.94042819436835));
#88007=CARTESIAN_POINT('',(640.,-11.0417504385235,-4.69890915568338));
#88008=CARTESIAN_POINT('Origin',(668.8,0.,0.));
#88009=CARTESIAN_POINT('Origin',(668.,0.,0.));
#88010=CARTESIAN_POINT('Origin',(669.6,0.,0.));
#88011=CARTESIAN_POINT('Origin',(668.,12.,0.));
#88012=CARTESIAN_POINT('Origin',(674.6,0.,0.));
#88013=CARTESIAN_POINT('Origin',(669.6,12.9,0.));
#88014=CARTESIAN_POINT('Origin',(640.,-9.14513292730969,-6.31242948430561));
#88015=CARTESIAN_POINT('',(640.,-9.29661268918755,-7.30088984352161));
#88016=CARTESIAN_POINT('',(640.,-10.1230748822772,-6.10355264807372));
#88017=CARTESIAN_POINT('Origin',(640.,-9.14513292730969,-6.31242948430561));
#88018=CARTESIAN_POINT('',(640.,-9.29661268918755,-7.30088984352161));
#88019=CARTESIAN_POINT('Ctrl Pts',(675.,-9.86502927874265,-7.00651106682565));
#88020=CARTESIAN_POINT('Ctrl Pts',(674.991906182189,-9.90272671607098,-6.96741155997444));
#88021=CARTESIAN_POINT('Ctrl Pts',(674.987834493111,-9.93733676924454,-6.92508679421849));
#88022=CARTESIAN_POINT('Ctrl Pts',(674.987834493111,-9.99889681716215,-6.83590166785504));
#88023=CARTESIAN_POINT('Ctrl Pts',(674.991906182189,-10.0261982666157,-6.78853213719756));
#88024=CARTESIAN_POINT('Ctrl Pts',(675.,-10.0493892450969,-6.73941954477757));
#88025=CARTESIAN_POINT('',(640.,-10.1230748822772,-6.10355264807372));
#88026=CARTESIAN_POINT('',(668.,-9.5963746723257,-7.20483123663183));
#88027=CARTESIAN_POINT('',(668.,-10.1395555887559,-6.41789782269309));
#88028=CARTESIAN_POINT('Origin',(668.,-9.14513292730969,-6.31242948430561));
#88029=CARTESIAN_POINT('',(669.6,-10.1395555887559,-6.41789782269309));
#88030=CARTESIAN_POINT('',(640.,-10.1395555887559,-6.4178978226931));
#88031=CARTESIAN_POINT('',(669.6,-9.5963746723257,-7.20483123663183));
#88032=CARTESIAN_POINT('Origin',(669.6,-9.14513292730969,-6.31242948430561));
#88033=CARTESIAN_POINT('',(640.,-9.59637467232571,-7.20483123663183));
#88034=CARTESIAN_POINT('Origin',(668.8,0.,0.));
#88035=CARTESIAN_POINT('Origin',(668.,0.,0.));
#88036=CARTESIAN_POINT('Origin',(669.6,0.,0.));
#88037=CARTESIAN_POINT('Origin',(668.,12.,0.));
#88038=CARTESIAN_POINT('Origin',(674.6,0.,0.));
#88039=CARTESIAN_POINT('Origin',(669.6,12.9,0.));
#88040=CARTESIAN_POINT('Origin',(640.,-7.36872872973994,-8.31757531736262));
#88041=CARTESIAN_POINT('',(640.,-7.2792527175532,-9.31356429483334));
#88042=CARTESIAN_POINT('',(640.,-8.36824096765044,-8.34880489096115));
#88043=CARTESIAN_POINT('Origin',(640.,-7.36872872973994,-8.31757531736262));
#88044=CARTESIAN_POINT('',(640.,-7.2792527175532,-9.31356429483334));
#88045=CARTESIAN_POINT('Ctrl Pts',(675.,-7.9016016065681,-9.16377062409794));
#88046=CARTESIAN_POINT('Ctrl Pts',(674.991906182189,-7.94756074933541,-9.13482886511152));
#88047=CARTESIAN_POINT('Ctrl Pts',(674.987834493111,-7.99129407669763,-9.10201670799259));
#88048=CARTESIAN_POINT('Ctrl Pts',(674.987834493111,-8.07240869926382,-9.03015542307488));
#88049=CARTESIAN_POINT('Ctrl Pts',(674.991906182189,-8.1102530889109,-8.99069602939965));
#88050=CARTESIAN_POINT('Ctrl Pts',(675.,-8.14452359238525,-8.9485605240776));
#88051=CARTESIAN_POINT('',(640.,-8.36824096765044,-8.34880489096115));
#88052=CARTESIAN_POINT('',(668.,-7.59329249157496,-9.29203471460322));
#88053=CARTESIAN_POINT('',(668.,-8.30901505047168,-8.65795985732407));
#88054=CARTESIAN_POINT('Origin',(668.,-7.36872872973994,-8.31757531736262));
#88055=CARTESIAN_POINT('',(669.6,-8.30901505047168,-8.65795985732407));
#88056=CARTESIAN_POINT('',(640.,-8.30901505047168,-8.65795985732407));
#88057=CARTESIAN_POINT('',(669.6,-7.59329249157496,-9.29203471460322));
#88058=CARTESIAN_POINT('Origin',(669.6,-7.36872872973994,-8.31757531736262));
#88059=CARTESIAN_POINT('',(640.,-7.59329249157496,-9.29203471460322));
#88060=CARTESIAN_POINT('Origin',(668.8,0.,0.));
#88061=CARTESIAN_POINT('Origin',(668.,0.,0.));
#88062=CARTESIAN_POINT('Origin',(669.6,0.,0.));
#88063=CARTESIAN_POINT('Origin',(668.,12.,0.));
#88064=CARTESIAN_POINT('Origin',(674.6,0.,0.));
#88065=CARTESIAN_POINT('Origin',(669.6,12.9,0.));
#88066=CARTESIAN_POINT('Origin',(640.,-5.16408080263683,-9.83933390613066));
#88067=CARTESIAN_POINT('',(640.,-4.83884903698172,-10.7849682427581));
#88068=CARTESIAN_POINT('',(640.,-6.12707530530208,-10.108854940257));
#88069=CARTESIAN_POINT('Origin',(640.,-5.16408080263683,-9.83933390613066));
#88070=CARTESIAN_POINT('',(640.,-4.83884903698172,-10.7849682427581));
#88071=CARTESIAN_POINT('Ctrl Pts',(675.,-5.47896157017303,-10.7884651416486));
#88072=CARTESIAN_POINT('Ctrl Pts',(674.991906182189,-5.53051144005636,-10.7713631203603));
#88073=CARTESIAN_POINT('Ctrl Pts',(674.987834493111,-5.58082641958515,-10.7499704951827));
#88074=CARTESIAN_POINT('Ctrl Pts',(674.987834493111,-5.67678152977605,-10.699609368385));
#88075=CARTESIAN_POINT('Ctrl Pts',(674.991906182189,-5.72296948124911,-10.6703533482234));
#88076=CARTESIAN_POINT('Ctrl Pts',(675.,-5.76632783262284,-10.6376436924123));
#88077=CARTESIAN_POINT('',(640.,-6.12707530530208,-10.108854940257));
#88078=CARTESIAN_POINT('',(668.,-5.14891575170907,-10.8392189101338));
#88079=CARTESIAN_POINT('',(668.,-5.99558475949487,-10.394852735451));
#88080=CARTESIAN_POINT('Origin',(668.,-5.16408080263683,-9.83933390613066));
#88081=CARTESIAN_POINT('',(669.6,-5.99558475949487,-10.394852735451));
#88082=CARTESIAN_POINT('',(640.,-5.99558475949487,-10.394852735451));
#88083=CARTESIAN_POINT('',(669.6,-5.14891575170907,-10.8392189101338));
#88084=CARTESIAN_POINT('Origin',(669.6,-5.16408080263683,-9.83933390613066));
#88085=CARTESIAN_POINT('',(640.,-5.14891575170908,-10.8392189101338));
#88086=CARTESIAN_POINT('Origin',(668.8,0.,0.));
#88087=CARTESIAN_POINT('Origin',(668.,0.,0.));
#88088=CARTESIAN_POINT('Origin',(669.6,0.,0.));
#88089=CARTESIAN_POINT('Origin',(668.,12.,0.));
#88090=CARTESIAN_POINT('Origin',(674.6,0.,0.));
#88091=CARTESIAN_POINT('Origin',(669.6,12.9,0.));
#88092=CARTESIAN_POINT('Origin',(640.,-2.65931526995444,-10.7892661727979));
#88093=CARTESIAN_POINT('',(640.,-2.11722903888146,-11.6295890381783));
#88094=CARTESIAN_POINT('',(640.,-3.52982629722213,-11.2814150846177));
#88095=CARTESIAN_POINT('Origin',(640.,-2.65931526995444,-10.7892661727979));
#88096=CARTESIAN_POINT('',(640.,-2.11722903888146,-11.6295890381783));
#88097=CARTESIAN_POINT('Ctrl Pts',(675.,-2.73790420253451,-11.7861732796419));
#88098=CARTESIAN_POINT('Ctrl Pts',(674.991906182189,-2.79204890847236,-11.7819049033656));
#88099=CARTESIAN_POINT('Ctrl Pts',(674.987834493111,-2.84602141644503,-11.7731750717457));
#88100=CARTESIAN_POINT('Ctrl Pts',(674.987834493111,-2.95124045203894,-11.7472409087023));
#88101=CARTESIAN_POINT('Ctrl Pts',(674.991906182189,-3.0030876894848,-11.7298885156047));
#88102=CARTESIAN_POINT('Ctrl Pts',(675.,-3.05301405897726,-11.7085056756055));
#88103=CARTESIAN_POINT('',(640.,-3.52982629722213,-11.2814150846177));
#88104=CARTESIAN_POINT('',(668.,-2.40530274390111,-11.7564671015651));
#88105=CARTESIAN_POINT('',(668.,-3.3337128753601,-11.5276345563458));
#88106=CARTESIAN_POINT('Origin',(668.,-2.65931526995444,-10.7892661727979));
#88107=CARTESIAN_POINT('',(669.6,-3.3337128753601,-11.5276345563458));
#88108=CARTESIAN_POINT('',(640.,-3.3337128753601,-11.5276345563458));
#88109=CARTESIAN_POINT('',(669.6,-2.40530274390111,-11.7564671015651));
#88110=CARTESIAN_POINT('Origin',(669.6,-2.65931526995444,-10.7892661727979));
#88111=CARTESIAN_POINT('',(640.,-2.40530274390111,-11.7564671015651));
#88112=CARTESIAN_POINT('Origin',(668.8,0.,0.));
#88113=CARTESIAN_POINT('Origin',(668.,0.,0.));
#88114=CARTESIAN_POINT('Origin',(669.6,0.,0.));
#88115=CARTESIAN_POINT('Origin',(668.,12.,0.));
#88116=CARTESIAN_POINT('Origin',(674.6,0.,0.));
#88117=CARTESIAN_POINT('Origin',(669.6,12.9,0.));
#88118=CARTESIAN_POINT('Origin',(640.,-8.40247638276174E-15,-11.112165506889));
#88119=CARTESIAN_POINT('',(640.,0.727436615144166,-11.7983403905358));
#88120=CARTESIAN_POINT('',(640.,-0.72743661514418,-11.7983403905358));
#88121=CARTESIAN_POINT('Origin',(640.,-8.40247638276174E-15,-11.112165506889));
#88122=CARTESIAN_POINT('',(640.,0.727436615144166,-11.7983403905358));
#88123=CARTESIAN_POINT('Ctrl Pts',(675.,0.162270205478472,-12.0989118676191));
#88124=CARTESIAN_POINT('Ctrl Pts',(674.991906182189,0.108677356987216,-12.1077251988691));
#88125=CARTESIAN_POINT('Ctrl Pts',(674.987834493111,0.0541840065519021,
-12.112165506889));
#88126=CARTESIAN_POINT('Ctrl Pts',(674.987834493111,-0.0541840065519376,
-12.112165506889));
#88127=CARTESIAN_POINT('Ctrl Pts',(674.991906182189,-0.108677356987223,
-12.1077251988691));
#88128=CARTESIAN_POINT('Ctrl Pts',(675.,-0.162270205478491,-12.0989118676191));
#88129=CARTESIAN_POINT('',(640.,-0.72743661514418,-11.7983403905358));
#88130=CARTESIAN_POINT('',(668.,0.47809771646265,-11.9904721580726));
#88131=CARTESIAN_POINT('',(668.,-0.478097716462668,-11.9904721580726));
#88132=CARTESIAN_POINT('Origin',(668.,-8.40247638276174E-15,-11.112165506889));
#88133=CARTESIAN_POINT('',(669.6,-0.478097716462668,-11.9904721580726));
#88134=CARTESIAN_POINT('',(640.,-0.478097716462663,-11.9904721580726));
#88135=CARTESIAN_POINT('',(669.6,0.47809771646265,-11.9904721580726));
#88136=CARTESIAN_POINT('Origin',(669.6,-8.40247638276174E-15,-11.112165506889));
#88137=CARTESIAN_POINT('',(640.,0.478097716462645,-11.9904721580726));
#88138=CARTESIAN_POINT('Origin',(668.8,0.,0.));
#88139=CARTESIAN_POINT('Origin',(668.,0.,0.));
#88140=CARTESIAN_POINT('Origin',(669.6,0.,0.));
#88141=CARTESIAN_POINT('Origin',(668.,12.,0.));
#88142=CARTESIAN_POINT('Origin',(674.6,0.,0.));
#88143=CARTESIAN_POINT('Origin',(669.6,12.9,0.));
#88144=CARTESIAN_POINT('Origin',(640.,2.65931526995443,-10.7892661727979));
#88145=CARTESIAN_POINT('',(640.,3.52982629722213,-11.2814150846177));
#88146=CARTESIAN_POINT('',(640.,2.11722903888144,-11.6295890381783));
#88147=CARTESIAN_POINT('Origin',(640.,2.65931526995443,-10.7892661727979));
#88148=CARTESIAN_POINT('',(640.,3.52982629722213,-11.2814150846177));
#88149=CARTESIAN_POINT('Ctrl Pts',(675.,3.05301405897724,-11.7085056756055));
#88150=CARTESIAN_POINT('Ctrl Pts',(674.991906182189,3.00308768948478,-11.7298885156048));
#88151=CARTESIAN_POINT('Ctrl Pts',(674.987834493111,2.95124045203896,-11.7472409087023));
#88152=CARTESIAN_POINT('Ctrl Pts',(674.987834493111,2.84602141644502,-11.7731750717457));
#88153=CARTESIAN_POINT('Ctrl Pts',(674.991906182189,2.79204890847233,-11.7819049033656));
#88154=CARTESIAN_POINT('Ctrl Pts',(675.,2.7379042025345,-11.7861732796419));
#88155=CARTESIAN_POINT('',(640.,2.11722903888144,-11.6295890381783));
#88156=CARTESIAN_POINT('',(668.,3.33371287536009,-11.5276345563458));
#88157=CARTESIAN_POINT('',(668.,2.40530274390109,-11.7564671015651));
#88158=CARTESIAN_POINT('Origin',(668.,2.65931526995443,-10.7892661727979));
#88159=CARTESIAN_POINT('',(669.6,2.40530274390109,-11.7564671015651));
#88160=CARTESIAN_POINT('',(640.,2.40530274390109,-11.7564671015651));
#88161=CARTESIAN_POINT('',(669.6,3.33371287536009,-11.5276345563458));
#88162=CARTESIAN_POINT('Origin',(669.6,2.65931526995443,-10.7892661727979));
#88163=CARTESIAN_POINT('',(640.,3.3337128753601,-11.5276345563458));
#88164=CARTESIAN_POINT('Origin',(668.8,0.,0.));
#88165=CARTESIAN_POINT('Origin',(668.,0.,0.));
#88166=CARTESIAN_POINT('Origin',(669.6,0.,0.));
#88167=CARTESIAN_POINT('Origin',(668.,12.,0.));
#88168=CARTESIAN_POINT('Origin',(674.6,0.,0.));
#88169=CARTESIAN_POINT('Origin',(669.6,12.9,0.));
#88170=CARTESIAN_POINT('Origin',(640.,5.16408080263683,-9.83933390613066));
#88171=CARTESIAN_POINT('',(640.,6.12707530530208,-10.108854940257));
#88172=CARTESIAN_POINT('',(640.,4.83884903698171,-10.7849682427581));
#88173=CARTESIAN_POINT('Origin',(640.,5.16408080263683,-9.83933390613066));
#88174=CARTESIAN_POINT('',(640.,6.12707530530208,-10.108854940257));
#88175=CARTESIAN_POINT('Ctrl Pts',(675.,5.76632783262284,-10.6376436924123));
#88176=CARTESIAN_POINT('Ctrl Pts',(674.991906182189,5.72296948124909,-10.6703533482234));
#88177=CARTESIAN_POINT('Ctrl Pts',(674.987834493111,5.67678152977605,-10.699609368385));
#88178=CARTESIAN_POINT('Ctrl Pts',(674.987834493111,5.58082641958514,-10.7499704951827));
#88179=CARTESIAN_POINT('Ctrl Pts',(674.991906182189,5.53051144005632,-10.7713631203603));
#88180=CARTESIAN_POINT('Ctrl Pts',(675.,5.47896157017303,-10.7884651416486));
#88181=CARTESIAN_POINT('',(640.,4.83884903698171,-10.7849682427581));
#88182=CARTESIAN_POINT('',(668.,5.99558475949487,-10.394852735451));
#88183=CARTESIAN_POINT('',(668.,5.14891575170907,-10.8392189101338));
#88184=CARTESIAN_POINT('Origin',(668.,5.16408080263683,-9.83933390613066));
#88185=CARTESIAN_POINT('',(669.6,5.14891575170907,-10.8392189101338));
#88186=CARTESIAN_POINT('',(640.,5.14891575170907,-10.8392189101338));
#88187=CARTESIAN_POINT('',(669.6,5.99558475949487,-10.394852735451));
#88188=CARTESIAN_POINT('Origin',(669.6,5.16408080263683,-9.83933390613066));
#88189=CARTESIAN_POINT('',(640.,5.99558475949487,-10.394852735451));
#88190=CARTESIAN_POINT('Origin',(668.8,0.,0.));
#88191=CARTESIAN_POINT('Origin',(668.,0.,0.));
#88192=CARTESIAN_POINT('Origin',(669.6,0.,0.));
#88193=CARTESIAN_POINT('Origin',(668.,12.,0.));
#88194=CARTESIAN_POINT('Origin',(674.6,0.,0.));
#88195=CARTESIAN_POINT('Origin',(669.6,12.9,0.));
#88196=CARTESIAN_POINT('Origin',(640.,7.36872872973994,-8.31757531736262));
#88197=CARTESIAN_POINT('',(640.,8.36824096765043,-8.34880489096116));
#88198=CARTESIAN_POINT('',(640.,7.2792527175532,-9.31356429483334));
#88199=CARTESIAN_POINT('Origin',(640.,7.36872872973994,-8.31757531736262));
#88200=CARTESIAN_POINT('',(640.,8.36824096765043,-8.34880489096116));
#88201=CARTESIAN_POINT('Ctrl Pts',(675.,8.14452359238524,-8.94856052407761));
#88202=CARTESIAN_POINT('Ctrl Pts',(674.991906182189,8.11025308891088,-8.99069602939967));
#88203=CARTESIAN_POINT('Ctrl Pts',(674.987834493111,8.07240869926381,-9.03015542307488));
#88204=CARTESIAN_POINT('Ctrl Pts',(674.987834493111,7.99129407669763,-9.10201670799259));
#88205=CARTESIAN_POINT('Ctrl Pts',(674.991906182189,7.94756074933537,-9.13482886511155));
#88206=CARTESIAN_POINT('Ctrl Pts',(675.,7.90160160656809,-9.16377062409795));
#88207=CARTESIAN_POINT('',(640.,7.2792527175532,-9.31356429483334));
#88208=CARTESIAN_POINT('',(668.,8.30901505047168,-8.65795985732408));
#88209=CARTESIAN_POINT('',(668.,7.59329249157495,-9.29203471460322));
#88210=CARTESIAN_POINT('Origin',(668.,7.36872872973994,-8.31757531736262));
#88211=CARTESIAN_POINT('',(669.6,7.59329249157495,-9.29203471460322));
#88212=CARTESIAN_POINT('',(640.,7.59329249157496,-9.29203471460322));
#88213=CARTESIAN_POINT('',(669.6,8.30901505047168,-8.65795985732408));
#88214=CARTESIAN_POINT('Origin',(669.6,7.36872872973994,-8.31757531736262));
#88215=CARTESIAN_POINT('',(640.,8.30901505047167,-8.65795985732408));
#88216=CARTESIAN_POINT('Origin',(668.8,0.,0.));
#88217=CARTESIAN_POINT('Origin',(668.,0.,0.));
#88218=CARTESIAN_POINT('Origin',(669.6,0.,0.));
#88219=CARTESIAN_POINT('Origin',(668.,12.,0.));
#88220=CARTESIAN_POINT('Origin',(674.6,0.,0.));
#88221=CARTESIAN_POINT('Origin',(669.6,12.9,0.));
#88222=CARTESIAN_POINT('Origin',(640.,9.14513292730969,-6.31242948430562));
#88223=CARTESIAN_POINT('',(640.,10.1230748822772,-6.10355264807372));
#88224=CARTESIAN_POINT('',(640.,9.29661268918755,-7.30088984352162));
#88225=CARTESIAN_POINT('Origin',(640.,9.14513292730969,-6.31242948430562));
#88226=CARTESIAN_POINT('',(640.,10.1230748822772,-6.10355264807372));
#88227=CARTESIAN_POINT('Ctrl Pts',(675.,10.0493892450969,-6.73941954477758));
#88228=CARTESIAN_POINT('Ctrl Pts',(674.991906182189,10.0261982666157,-6.78853213719754));
#88229=CARTESIAN_POINT('Ctrl Pts',(674.987834493111,9.99889681716214,-6.83590166785507));
#88230=CARTESIAN_POINT('Ctrl Pts',(674.987834493111,9.93733676924454,-6.92508679421849));
#88231=CARTESIAN_POINT('Ctrl Pts',(674.991906182189,9.90272671607097,-6.96741155997445));
#88232=CARTESIAN_POINT('Ctrl Pts',(675.,9.86502927874264,-7.00651106682565));
#88233=CARTESIAN_POINT('',(640.,9.29661268918755,-7.30088984352162));
#88234=CARTESIAN_POINT('',(668.,10.1395555887559,-6.4178978226931));
#88235=CARTESIAN_POINT('',(668.,9.5963746723257,-7.20483123663184));
#88236=CARTESIAN_POINT('Origin',(668.,9.14513292730969,-6.31242948430562));
#88237=CARTESIAN_POINT('',(669.6,9.5963746723257,-7.20483123663184));
#88238=CARTESIAN_POINT('',(640.,9.5963746723257,-7.20483123663184));
#88239=CARTESIAN_POINT('',(669.6,10.1395555887559,-6.4178978226931));
#88240=CARTESIAN_POINT('Origin',(669.6,9.14513292730969,-6.31242948430562));
#88241=CARTESIAN_POINT('',(640.,10.1395555887559,-6.4178978226931));
#88242=CARTESIAN_POINT('Origin',(668.8,0.,0.));
#88243=CARTESIAN_POINT('Origin',(668.,0.,0.));
#88244=CARTESIAN_POINT('Origin',(669.6,0.,0.));
#88245=CARTESIAN_POINT('Origin',(668.,12.,0.));
#88246=CARTESIAN_POINT('Origin',(674.6,0.,0.));
#88247=CARTESIAN_POINT('Origin',(669.6,12.9,0.));
#88248=CARTESIAN_POINT('Origin',(640.,11.0311453091351,-1.33942354064812));
#88249=CARTESIAN_POINT('',(640.,11.8,-0.7));
#88250=CARTESIAN_POINT('',(640.,11.6246344106287,-2.14426556639496));
#88251=CARTESIAN_POINT('Origin',(640.,11.0311453091351,-1.33942354064812));
#88252=CARTESIAN_POINT('',(640.,11.8,-0.7));
#88253=CARTESIAN_POINT('Ctrl Pts',(675.,12.0302566897885,-1.2972755982442));
#88254=CARTESIAN_POINT('Ctrl Pts',(674.991906182189,12.0325458578882,-1.35154002422057));
#88255=CARTESIAN_POINT('Ctrl Pts',(674.987834493111,12.0303853435058,-1.40617127676511));
#88256=CARTESIAN_POINT('Ctrl Pts',(674.987834493111,12.0173230229604,-1.51374916504179));
#88257=CARTESIAN_POINT('Ctrl Pts',(674.991906182189,12.0063466422278,-1.56730997761024));
#88258=CARTESIAN_POINT('Ctrl Pts',(675.,11.991137666043,-1.61944974420488));
#88259=CARTESIAN_POINT('',(640.,11.6246344106287,-2.14426556639496));
#88260=CARTESIAN_POINT('',(668.,11.9606764275243,-0.970679862809454));
#88261=CARTESIAN_POINT('',(668.,11.8454198043642,-1.91990355444645));
#88262=CARTESIAN_POINT('Origin',(668.,11.0311453091351,-1.33942354064812));
#88263=CARTESIAN_POINT('',(669.6,11.8454198043642,-1.91990355444645));
#88264=CARTESIAN_POINT('',(640.,11.8454198043642,-1.91990355444646));
#88265=CARTESIAN_POINT('',(669.6,11.9606764275243,-0.970679862809454));
#88266=CARTESIAN_POINT('Origin',(669.6,11.0311453091351,-1.33942354064812));
#88267=CARTESIAN_POINT('',(640.,11.9606764275243,-0.970679862809442));
#88268=CARTESIAN_POINT('Origin',(674.6,0.,0.));
#88269=CARTESIAN_POINT('Origin',(668.8,0.,0.));
#88270=CARTESIAN_POINT('Origin',(668.,0.,0.));
#88271=CARTESIAN_POINT('Origin',(669.6,0.,0.));
#88272=CARTESIAN_POINT('Origin',(668.,12.,0.));
#88273=CARTESIAN_POINT('Origin',(640.,10.3900552403499,-3.94042819436836));
#88274=CARTESIAN_POINT('',(640.,11.2895924806261,-3.50358411079143));
#88275=CARTESIAN_POINT('',(640.,10.7736873231385,-4.86391421215923));
#88276=CARTESIAN_POINT('Origin',(640.,10.3900552403499,-3.94042819436836));
#88277=CARTESIAN_POINT('',(640.,11.2895924806261,-3.50358411079143));
#88278=CARTESIAN_POINT('Ctrl Pts',(675.,11.3702209229272,-4.13860799832839));
#88279=CARTESIAN_POINT('Ctrl Pts',(674.991906182189,11.3594572448126,-4.19184343249188));
#88280=CARTESIAN_POINT('Ctrl Pts',(674.987834493111,11.3442853965581,-4.24437015519106));
#88281=CARTESIAN_POINT('Ctrl Pts',(674.987834493111,11.3058575695124,-4.34569600763074));
#88282=CARTESIAN_POINT('Ctrl Pts',(674.991906182189,11.2823822010156,-4.39507362048222));
#88283=CARTESIAN_POINT('Ctrl Pts',(675.,11.2551373071591,-4.44205855398095));
#88284=CARTESIAN_POINT('',(640.,10.7736873231385,-4.86391421215923));
#88285=CARTESIAN_POINT('',(668.,11.3808220120066,-3.80485089471661));
#88286=CARTESIAN_POINT('',(668.,11.0417504385235,-4.69890915568339));
#88287=CARTESIAN_POINT('Origin',(668.,10.3900552403499,-3.94042819436836));
#88288=CARTESIAN_POINT('',(669.6,11.0417504385235,-4.69890915568339));
#88289=CARTESIAN_POINT('',(640.,11.0417504385235,-4.69890915568339));
#88290=CARTESIAN_POINT('',(669.6,11.3808220120066,-3.80485089471661));
#88291=CARTESIAN_POINT('Origin',(669.6,10.3900552403499,-3.94042819436836));
#88292=CARTESIAN_POINT('',(640.,11.3808220120066,-3.80485089471661));
#88293=CARTESIAN_POINT('Origin',(668.8,0.,0.));
#88294=CARTESIAN_POINT('Origin',(668.,0.,0.));
#88295=CARTESIAN_POINT('Origin',(669.6,0.,0.));
#88296=CARTESIAN_POINT('Origin',(668.,12.,0.));
#88297=CARTESIAN_POINT('Origin',(639.,0.,0.));
#88298=CARTESIAN_POINT('',(640.,-1.56754790290861E-15,12.8));
#88299=CARTESIAN_POINT('Origin',(640.,0.,0.));
#88300=CARTESIAN_POINT('',(639.,-1.69001258282335E-15,13.8));
#88301=CARTESIAN_POINT('Origin',(639.,-1.56754790290861E-15,12.8));
#88302=CARTESIAN_POINT('',(639.,-13.8,-1.69001258282335E-15));
#88303=CARTESIAN_POINT('Origin',(639.,0.,0.));
#88304=CARTESIAN_POINT('Origin',(639.,0.,0.));
#88305=CARTESIAN_POINT('Origin',(640.,0.,0.));
#88306=CARTESIAN_POINT('Origin',(639.994987437107,0.,0.));
#88307=CARTESIAN_POINT('Origin',(640.,12.9,0.));
#88308=CARTESIAN_POINT('Origin',(640.,0.,0.));
#88309=CARTESIAN_POINT('',(640.,11.8,0.7));
#88310=CARTESIAN_POINT('',(640.,11.6246344106287,-2.14426556639496));
#88311=CARTESIAN_POINT('',(640.,10.7736873231385,-4.86391421215923));
#88312=CARTESIAN_POINT('',(640.,9.29661268918755,-7.30088984352162));
#88313=CARTESIAN_POINT('',(640.,7.2792527175532,-9.31356429483334));
#88314=CARTESIAN_POINT('',(640.,4.83884903698171,-10.7849682427581));
#88315=CARTESIAN_POINT('',(640.,2.11722903888144,-11.6295890381783));
#88316=CARTESIAN_POINT('',(640.,-0.72743661514418,-11.7983403905358));
#88317=CARTESIAN_POINT('',(640.,-3.52982629722213,-11.2814150846177));
#88318=CARTESIAN_POINT('',(640.,-6.12707530530208,-10.108854940257));
#88319=CARTESIAN_POINT('',(640.,-8.36824096765044,-8.34880489096115));
#88320=CARTESIAN_POINT('',(640.,-10.1230748822772,-6.10355264807372));
#88321=CARTESIAN_POINT('',(640.,-11.2895924806261,-3.50358411079141));
#88322=CARTESIAN_POINT('',(640.,-11.8,-0.699999999999999));
#88323=CARTESIAN_POINT('',(640.,-11.6246344106287,2.14426556639495));
#88324=CARTESIAN_POINT('',(640.,-10.7736873231385,4.86391421215922));
#88325=CARTESIAN_POINT('',(640.,-9.29661268918755,7.30088984352162));
#88326=CARTESIAN_POINT('',(640.,-7.2792527175532,9.31356429483334));
#88327=CARTESIAN_POINT('',(640.,-4.83884903698171,10.7849682427581));
#88328=CARTESIAN_POINT('',(640.,-2.11722903888145,11.6295890381783));
#88329=CARTESIAN_POINT('',(640.,0.727436615144177,11.7983403905358));
#88330=CARTESIAN_POINT('',(640.,3.52982629722213,11.2814150846177));
#88331=CARTESIAN_POINT('',(640.,6.12707530530208,10.108854940257));
#88332=CARTESIAN_POINT('',(640.,8.36824096765044,8.34880489096115));
#88333=CARTESIAN_POINT('',(640.,10.1230748822772,6.10355264807372));
#88334=CARTESIAN_POINT('',(640.,11.2895924806261,3.50358411079142));
#88335=CARTESIAN_POINT('Origin',(627.,0.,0.));
#88336=CARTESIAN_POINT('',(627.,-13.8,-1.69001258282335E-15));
#88337=CARTESIAN_POINT('Origin',(674.6,0.,0.));
#88338=CARTESIAN_POINT('Origin',(640.,11.6246344106287,-2.14426556639496));
#88339=CARTESIAN_POINT('Origin',(669.6,12.9,0.));
#88340=CARTESIAN_POINT('Origin',(640.,10.7736873231385,-4.86391421215923));
#88341=CARTESIAN_POINT('Origin',(640.,9.29661268918755,-7.30088984352162));
#88342=CARTESIAN_POINT('Origin',(640.,7.2792527175532,-9.31356429483334));
#88343=CARTESIAN_POINT('Origin',(640.,4.83884903698171,-10.7849682427581));
#88344=CARTESIAN_POINT('Origin',(640.,2.11722903888144,-11.6295890381783));
#88345=CARTESIAN_POINT('Origin',(640.,-0.72743661514418,-11.7983403905358));
#88346=CARTESIAN_POINT('Origin',(640.,-3.52982629722213,-11.2814150846177));
#88347=CARTESIAN_POINT('Origin',(640.,-6.12707530530208,-10.108854940257));
#88348=CARTESIAN_POINT('Origin',(640.,-8.36824096765044,-8.34880489096115));
#88349=CARTESIAN_POINT('Origin',(640.,-10.1230748822772,-6.10355264807372));
#88350=CARTESIAN_POINT('Origin',(640.,-11.2895924806261,-3.50358411079141));
#88351=CARTESIAN_POINT('Origin',(640.,-11.8,-0.699999999999999));
#88352=CARTESIAN_POINT('Origin',(640.,-11.6246344106287,2.14426556639495));
#88353=CARTESIAN_POINT('Origin',(640.,-10.7736873231385,4.86391421215922));
#88354=CARTESIAN_POINT('Origin',(640.,-9.29661268918755,7.30088984352162));
#88355=CARTESIAN_POINT('Origin',(640.,-7.2792527175532,9.31356429483334));
#88356=CARTESIAN_POINT('Origin',(640.,-4.83884903698171,10.7849682427581));
#88357=CARTESIAN_POINT('Origin',(640.,-2.11722903888145,11.6295890381783));
#88358=CARTESIAN_POINT('Origin',(640.,0.727436615144177,11.7983403905358));
#88359=CARTESIAN_POINT('Origin',(640.,3.52982629722213,11.2814150846177));
#88360=CARTESIAN_POINT('Origin',(640.,6.12707530530208,10.108854940257));
#88361=CARTESIAN_POINT('Origin',(640.,8.36824096765044,8.34880489096115));
#88362=CARTESIAN_POINT('Origin',(640.,10.1230748822772,6.10355264807372));
#88363=CARTESIAN_POINT('Origin',(640.,11.2895924806261,3.50358411079142));
#88364=CARTESIAN_POINT('Origin',(654.,0.,0.));
#88365=CARTESIAN_POINT('Origin',(640.,11.8,0.7));
#88366=CARTESIAN_POINT('Origin',(565.,22.5,38.9711431702997));
#88367=CARTESIAN_POINT('Origin',(565.,22.5,-38.9711431702997));
#88368=CARTESIAN_POINT('Origin',(552.,0.,0.));
#88369=CARTESIAN_POINT('Origin',(552.,-10.5,18.1865334794732));
#88370=CARTESIAN_POINT('Origin',(497.,-10.5,18.1865334794732));
#88371=CARTESIAN_POINT('Origin',(571.,0.,0.));
#88372=CARTESIAN_POINT('',(571.,-32.,-3.91886975727153E-15));
#88373=CARTESIAN_POINT('Origin',(669.6,12.9,0.));
#90350=UNCERTAINTY_MEASURE_WITH_UNIT(LENGTH_MEASURE(0.01),#90375,
'DISTANCE_ACCURACY_VALUE',
'Maximum model space distance between geometric entities at asserted c
onnectivities');
#90355=UNCERTAINTY_MEASURE_WITH_UNIT(LENGTH_MEASURE(0.01),#90375,
'DISTANCE_ACCURACY_VALUE',
'Maximum model space distance between geometric entities at asserted c
onnectivities');
#90369=(
GEOMETRIC_REPRESENTATION_CONTEXT(3)
GLOBAL_UNCERTAINTY_ASSIGNED_CONTEXT((#90350))
GLOBAL_UNIT_ASSIGNED_CONTEXT((#90375,#90377,#90378))
REPRESENTATION_CONTEXT('','3D')
);
#90374=(
GEOMETRIC_REPRESENTATION_CONTEXT(3)
GLOBAL_UNCERTAINTY_ASSIGNED_CONTEXT((#90355))
GLOBAL_UNIT_ASSIGNED_CONTEXT((#90375,#90377,#90378))
REPRESENTATION_CONTEXT('','3D')
);
#90375=(
LENGTH_UNIT()
NAMED_UNIT(*)
SI_UNIT(.MILLI.,.METRE.)
);
#90377=(
NAMED_UNIT(*)
PLANE_ANGLE_UNIT()
SI_UNIT($,.RADIAN.)
);
#90378=(
NAMED_UNIT(*)
SI_UNIT($,.STERADIAN.)
SOLID_ANGLE_UNIT()
);
#90392=SHAPE_DEFINITION_REPRESENTATION(#90410,#90453);
#90410=PRODUCT_DEFINITION_SHAPE('',$,#90472);
#90453=SHAPE_REPRESENTATION('',(#44271),#90369);
#90458=PRODUCT_DEFINITION_CONTEXT('part definition',#90514,'design');
#90472=PRODUCT_DEFINITION('2026-10-11-12-53-13-263',
'13_Inner_Tripod_Housing_with_Stub',#90490,#90458);
#90490=PRODUCT_DEFINITION_FORMATION('',$,#90529);
#90514=APPLICATION_CONTEXT(
'Core Data for Automotive Mechanical Design Process');
#90515=PRODUCT_CONTEXT('part definition',#90514,'mechanical');
#90529=PRODUCT('2026-10-11-12-53-13-263',
'13_Inner_Tripod_Housing_with_Stub',$,(#90515));
#90660=COLOUR_RGB('Dark Blue',0.08,0.2,0.34);
#90661=FILL_AREA_STYLE_COLOUR('',#90660);
#90662=FILL_AREA_STYLE('',(#90661));
#90663=SURFACE_STYLE_FILL_AREA(#90662);
#90664=SURFACE_SIDE_STYLE('',(#90663));
#90665=SURFACE_STYLE_USAGE(.BOTH.,#90664);
#90666=PRESENTATION_STYLE_ASSIGNMENT((#90665));
ENDSEC;
END-ISO-10303-21;
